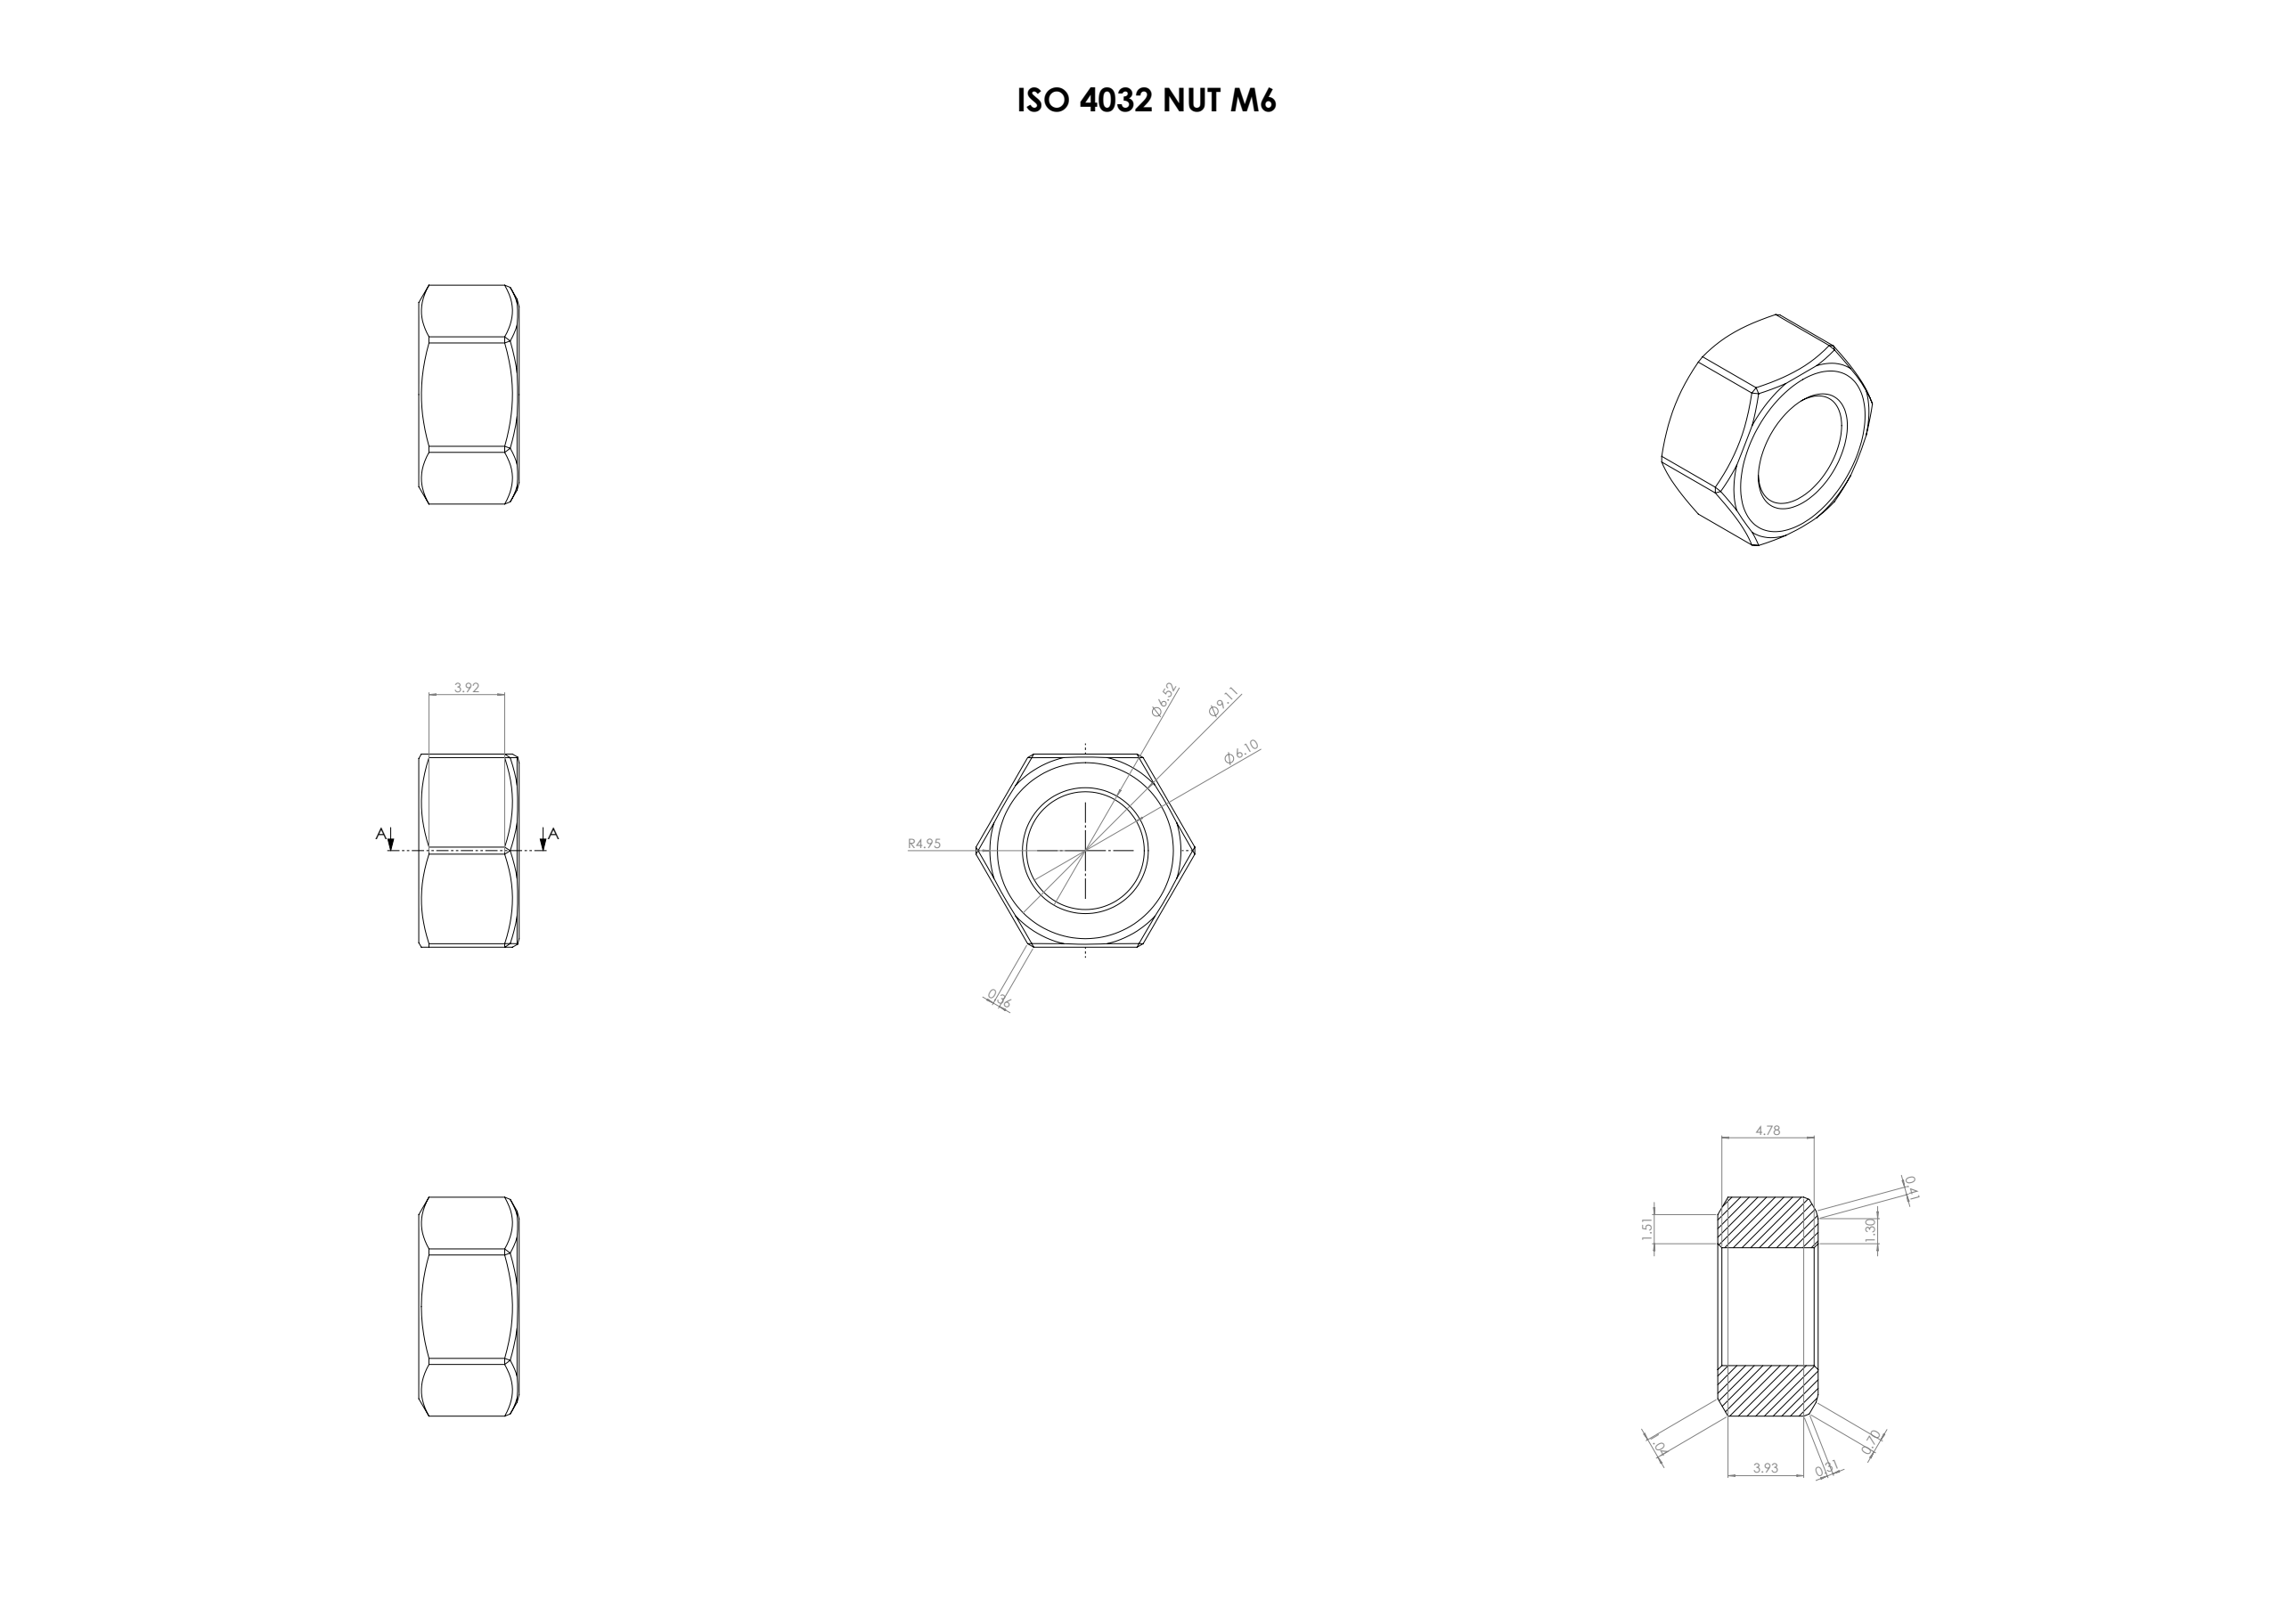
ISO-10303-21;
HEADER;
/* Generated by software containing ST-Developer
 * from STEP Tools, Inc. (www.steptools.com) 
 */

FILE_DESCRIPTION(
/* description */ (''),
/* implementation_level */ '2;1');

FILE_NAME(
/* name */ '08_ISO_4032_Nut_M6.step',
/* time_stamp */ '2026-10-21T02:03:06-07:00',
/* author */ (''),
/* organization */ (''),
/* preprocessor_version */ 'ST-DEVELOPER v20.2',
/* originating_system */ 'Autodesk Translation Framework v15.15.0.0',
/* authorisation */ '');

FILE_SCHEMA (('AUTOMOTIVE_DESIGN { 1 0 10303 214 3 1 1 }'));
ENDSEC;

DATA;
#10=MECHANICAL_DESIGN_GEOMETRIC_PRESENTATION_REPRESENTATION('',(#122),#38528);
#80=B_SPLINE_SURFACE_WITH_KNOTS('',3,3,((#33437,#33438,#33439,#33440,#33441),
(#33442,#33443,#33444,#33445,#33446),(#33447,#33448,#33449,#33450,#33451),
(#33452,#33453,#33454,#33455,#33456)),.UNSPECIFIED.,.F.,.F.,.F.,(4,4),(4,
1,4),(0.,1.),(0.0610870649866808,0.309114526274187,0.639817807990862),
 .UNSPECIFIED.);
#81=B_SPLINE_SURFACE_WITH_KNOTS('',3,3,((#33486,#33487,#33488,#33489,#33490),
(#33491,#33492,#33493,#33494,#33495),(#33496,#33497,#33498,#33499,#33500),
(#33501,#33502,#33503,#33504,#33505)),.UNSPECIFIED.,.F.,.F.,.F.,(4,4),(4,
1,4),(0.,1.),(0.0610870649866807,0.309114526274187,0.639817807990862),
 .UNSPECIFIED.);
#82=B_SPLINE_SURFACE_WITH_KNOTS('',3,3,((#33575,#33576,#33577,#33578,#33579),
(#33580,#33581,#33582,#33583,#33584),(#33585,#33586,#33587,#33588,#33589),
(#33590,#33591,#33592,#33593,#33594)),.UNSPECIFIED.,.F.,.F.,.F.,(4,4),(4,
1,4),(0.,1.),(0.061087064986681,0.309114526274187,0.639817807990862),
 .UNSPECIFIED.);
#83=B_SPLINE_SURFACE_WITH_KNOTS('',3,3,((#33668,#33669,#33670,#33671,#33672),
(#33673,#33674,#33675,#33676,#33677),(#33678,#33679,#33680,#33681,#33682),
(#33683,#33684,#33685,#33686,#33687)),.UNSPECIFIED.,.F.,.F.,.F.,(4,4),(4,
1,4),(0.,1.),(0.0610870649866801,0.309114526274187,0.639817807990862),
 .UNSPECIFIED.);
#84=B_SPLINE_SURFACE_WITH_KNOTS('',3,3,((#33701,#33702,#33703,#33704,#33705),
(#33706,#33707,#33708,#33709,#33710),(#33711,#33712,#33713,#33714,#33715),
(#33716,#33717,#33718,#33719,#33720)),.UNSPECIFIED.,.F.,.F.,.F.,(4,4),(4,
1,4),(0.,1.),(0.0610870649866807,0.391790346703356,0.639817807990862),
 .UNSPECIFIED.);
#85=B_SPLINE_SURFACE_WITH_KNOTS('',3,3,((#33742,#33743,#33744,#33745,#33746),
(#33747,#33748,#33749,#33750,#33751),(#33752,#33753,#33754,#33755,#33756),
(#33757,#33758,#33759,#33760,#33761)),.UNSPECIFIED.,.F.,.F.,.F.,(4,4),(4,
1,4),(0.,1.),(0.0610870649866804,0.309114526274187,0.639817807990861),
 .UNSPECIFIED.);
#98=SHAPE_REPRESENTATION_RELATIONSHIP('SRR','None',#38583,#110);
#110=ADVANCED_BREP_SHAPE_REPRESENTATION('',(#134),#38523);
#122=STYLED_ITEM('',(#38713),#134);
#134=MANIFOLD_SOLID_BREP('Body1',#17079);
#385=CYLINDRICAL_SURFACE('',#18726,3.05);
#719=B_SPLINE_CURVE_WITH_KNOTS('',3,(#33230,#33231,#33232,#33233,#33234,
#33235,#33236,#33237,#33238,#33239,#33240,#33241,#33242,#33243,#33244,#33245,
#33246,#33247,#33248),.UNSPECIFIED.,.F.,.F.,(4,3,3,3,3,3,4),(-0.113329393083273,
-0.0991044193051623,-0.0674458844185764,-0.061631000326846,-0.0331038403136512,
-0.00584534044920819,0.),.UNSPECIFIED.);
#720=B_SPLINE_CURVE_WITH_KNOTS('',3,(#33252,#33253,#33254,#33255,#33256,
#33257,#33258,#33259,#33260,#33261,#33262,#33263,#33264,#33265,#33266,#33267,
#33268,#33269,#33270,#33271,#33272,#33273,#33274,#33275,#33276,#33277,#33278,
#33279,#33280,#33281,#33282),.UNSPECIFIED.,.F.,.F.,(4,3,3,3,3,3,3,3,3,3,
4),(-0.226650511587635,-0.198574388081722,-0.170498264575808,-0.13944012666617,
-0.131476509591221,-0.0991044193051576,-0.0762723334429418,-0.0616310003268515,
-0.0331662800001561,-0.00604790654757715,0.),.UNSPECIFIED.);
#721=B_SPLINE_CURVE_WITH_KNOTS('',3,(#33286,#33287,#33288,#33289,#33290,
#33291,#33292,#33293,#33294,#33295,#33296,#33297,#33298,#33299,#33300,#33301,
#33302,#33303,#33304,#33305,#33306,#33307,#33308,#33309,#33310,#33311,#33312,
#33313,#33314,#33315,#33316),.UNSPECIFIED.,.F.,.F.,(4,3,3,3,3,3,3,3,3,3,
4),(-0.226650511587582,-0.198574388081676,-0.170498264575771,-0.13944012666705,
-0.131476509591215,-0.0991044193051536,-0.0762723334429342,-0.0616310003268419,
-0.0331662799998172,-0.00604790654743552,0.),.UNSPECIFIED.);
#722=B_SPLINE_CURVE_WITH_KNOTS('',3,(#33320,#33321,#33322,#33323,#33324,
#33325,#33326,#33327,#33328,#33329,#33330,#33331,#33332,#33333,#33334,#33335,
#33336,#33337,#33338,#33339,#33340,#33341,#33342,#33343,#33344,#33345,#33346,
#33347,#33348,#33349,#33350),.UNSPECIFIED.,.F.,.F.,(4,3,3,3,3,3,3,3,3,3,
4),(-0.226650511587584,-0.198574388081659,-0.170498264575734,-0.139440596738821,
-0.131476509591163,-0.0991044193051282,-0.0762723334429448,-0.0616310003268502,
-0.0331645723826234,-0.00604411953936661,0.),.UNSPECIFIED.);
#723=B_SPLINE_CURVE_WITH_KNOTS('',3,(#33354,#33355,#33356,#33357,#33358,
#33359,#33360,#33361,#33362,#33363,#33364,#33365,#33366,#33367,#33368,#33369,
#33370,#33371,#33372,#33373,#33374,#33375,#33376,#33377,#33378,#33379,#33380,
#33381,#33382,#33383,#33384),.UNSPECIFIED.,.F.,.F.,(4,3,3,3,3,3,3,3,3,3,
4),(-0.226650511587706,-0.198574388081775,-0.170498264575844,-0.139440126665696,
-0.131476509591268,-0.0991044193051773,-0.0762723334429522,-0.0616310003268415,
-0.0331662800006236,-0.00604790654845245,0.),.UNSPECIFIED.);
#724=B_SPLINE_CURVE_WITH_KNOTS('',3,(#33388,#33389,#33390,#33391,#33392,
#33393,#33394,#33395,#33396,#33397,#33398,#33399,#33400,#33401,#33402,#33403,
#33404,#33405,#33406,#33407,#33408,#33409,#33410,#33411,#33412,#33413,#33414,
#33415,#33416,#33417,#33418),.UNSPECIFIED.,.F.,.F.,(4,3,3,3,3,3,3,3,3,3,
4),(-0.226650511587727,-0.198574388081779,-0.170498264575831,-0.139440126665785,
-0.13147650959124,-0.0991044193051654,-0.0762723334429508,-0.0616310003268513,
-0.0331662799998889,-0.00604790654758933,0.),.UNSPECIFIED.);
#725=B_SPLINE_CURVE_WITH_KNOTS('',3,(#33421,#33422,#33423,#33424,#33425,
#33426,#33427,#33428,#33429,#33430,#33431,#33432,#33433,#33434,#33435,#33436),
 .UNSPECIFIED.,.F.,.F.,(4,3,3,3,3,4),(-0.226650511587688,-0.198574388081761,
-0.170498264575834,-0.150386414929284,-0.131476509591241,-0.113329393083273),
 .UNSPECIFIED.);
#726=B_SPLINE_CURVE_WITH_KNOTS('',3,(#33458,#33459,#33460,#33461),
 .UNSPECIFIED.,.F.,.F.,(4,4),(0.474834937773607,0.639817807990862),
 .UNSPECIFIED.);
#727=B_SPLINE_CURVE_WITH_KNOTS('',3,(#33463,#33464,#33465,#33466,#33467,
#33468),.UNSPECIFIED.,.F.,.F.,(4,2,4),(-0.0356915196979304,-0.0178436364936306,
0.),.UNSPECIFIED.);
#728=B_SPLINE_CURVE_WITH_KNOTS('',3,(#33470,#33471,#33472,#33473,#33474),
 .UNSPECIFIED.,.F.,.F.,(4,1,4),(-0.63803777562903,-0.309114526274187,-0.0628670973485611),
 .UNSPECIFIED.);
#729=B_SPLINE_CURVE_WITH_KNOTS('',3,(#33476,#33477,#33478,#33479,#33480,
#33481),.UNSPECIFIED.,.F.,.F.,(4,2,4),(-0.035691517766977,-0.0178476663798058,
0.),.UNSPECIFIED.);
#730=B_SPLINE_CURVE_WITH_KNOTS('',3,(#33482,#33483,#33484,#33485),
 .UNSPECIFIED.,.F.,.F.,(4,4),(0.0610870649866808,0.226069935203935),
 .UNSPECIFIED.);
#731=B_SPLINE_CURVE_WITH_KNOTS('',3,(#33507,#33508,#33509,#33510),
 .UNSPECIFIED.,.F.,.F.,(4,4),(0.474834937773608,0.639817807990862),
 .UNSPECIFIED.);
#732=B_SPLINE_CURVE_WITH_KNOTS('',3,(#33512,#33513,#33514,#33515,#33516,
#33517),.UNSPECIFIED.,.F.,.F.,(4,2,4),(-0.0356915197043745,-0.0178436364953559,
0.),.UNSPECIFIED.);
#733=B_SPLINE_CURVE_WITH_KNOTS('',3,(#33519,#33520,#33521,#33522,#33523),
 .UNSPECIFIED.,.F.,.F.,(4,1,4),(-0.638037775629031,-0.309114526274187,-0.062867097348561),
 .UNSPECIFIED.);
#734=B_SPLINE_CURVE_WITH_KNOTS('',3,(#33524,#33525,#33526,#33527,#33528,
#33529),.UNSPECIFIED.,.F.,.F.,(4,2,4),(-0.0356915177684809,-0.0178476663801996,
0.),.UNSPECIFIED.);
#735=B_SPLINE_CURVE_WITH_KNOTS('',3,(#33530,#33531,#33532,#33533),
 .UNSPECIFIED.,.F.,.F.,(4,4),(0.0610870649866807,0.226069935203935),
 .UNSPECIFIED.);
#736=B_SPLINE_CURVE_WITH_KNOTS('',3,(#33536,#33537,#33538,#33539),
 .UNSPECIFIED.,.F.,.F.,(4,4),(0.061087064986681,0.226069935203935),
 .UNSPECIFIED.);
#737=B_SPLINE_CURVE_WITH_KNOTS('',3,(#33542,#33543,#33544,#33545),
 .UNSPECIFIED.,.F.,.F.,(4,4),(0.0610870649866804,0.226069935203935),
 .UNSPECIFIED.);
#738=B_SPLINE_CURVE_WITH_KNOTS('',3,(#33546,#33547,#33548,#33549),
 .UNSPECIFIED.,.F.,.F.,(4,4),(0.474834937773607,0.639817807990862),
 .UNSPECIFIED.);
#739=B_SPLINE_CURVE_WITH_KNOTS('',3,(#33552,#33553,#33554,#33555),
 .UNSPECIFIED.,.F.,.F.,(4,4),(0.0610870649866807,0.226069935203935),
 .UNSPECIFIED.);
#740=B_SPLINE_CURVE_WITH_KNOTS('',3,(#33556,#33557,#33558,#33559),
 .UNSPECIFIED.,.F.,.F.,(4,4),(0.474834937773607,0.639817807990861),
 .UNSPECIFIED.);
#741=B_SPLINE_CURVE_WITH_KNOTS('',3,(#33562,#33563,#33564,#33565),
 .UNSPECIFIED.,.F.,.F.,(4,4),(0.0610870649866801,0.226069935203935),
 .UNSPECIFIED.);
#742=B_SPLINE_CURVE_WITH_KNOTS('',3,(#33566,#33567,#33568,#33569),
 .UNSPECIFIED.,.F.,.F.,(4,4),(0.474834937773608,0.639817807990862),
 .UNSPECIFIED.);
#743=B_SPLINE_CURVE_WITH_KNOTS('',3,(#33571,#33572,#33573,#33574),
 .UNSPECIFIED.,.F.,.F.,(4,4),(0.474834937773608,0.639817807990862),
 .UNSPECIFIED.);
#744=B_SPLINE_CURVE_WITH_KNOTS('',3,(#33596,#33597,#33598,#33599,#33600,
#33601),.UNSPECIFIED.,.F.,.F.,(4,2,4),(-0.0356915197030877,-0.0178436364955222,
0.),.UNSPECIFIED.);
#745=B_SPLINE_CURVE_WITH_KNOTS('',3,(#33603,#33604,#33605,#33606,#33607),
 .UNSPECIFIED.,.F.,.F.,(4,1,4),(-0.63803777562903,-0.309114526274187,-0.0628670973485611),
 .UNSPECIFIED.);
#746=B_SPLINE_CURVE_WITH_KNOTS('',3,(#33608,#33609,#33610,#33611,#33612,
#33613),.UNSPECIFIED.,.F.,.F.,(4,2,4),(-0.0356915177637329,-0.0178476663792099,
0.),.UNSPECIFIED.);
#747=B_SPLINE_CURVE_WITH_KNOTS('',3,(#33618,#33619,#33620,#33621,#33622,
#33623),.UNSPECIFIED.,.F.,.F.,(4,2,4),(-0.0356915177685627,-0.0178476663800234,
0.),.UNSPECIFIED.);
#748=B_SPLINE_CURVE_WITH_KNOTS('',3,(#33629,#33630,#33631,#33632,#33633,
#33634),.UNSPECIFIED.,.F.,.F.,(4,2,4),(-0.035691519698345,-0.0178436364936918,
0.),.UNSPECIFIED.);
#749=B_SPLINE_CURVE_WITH_KNOTS('',3,(#33636,#33637,#33638,#33639,#33640,
#33641),.UNSPECIFIED.,.F.,.F.,(4,2,4),(-0.0356915177661021,-0.0178476663801455,
0.),.UNSPECIFIED.);
#750=B_SPLINE_CURVE_WITH_KNOTS('',3,(#33646,#33647,#33648,#33649,#33650,
#33651),.UNSPECIFIED.,.F.,.F.,(4,2,4),(-0.0356915197010578,-0.0178436364947975,
0.),.UNSPECIFIED.);
#751=B_SPLINE_CURVE_WITH_KNOTS('',3,(#33654,#33655,#33656,#33657,#33658,
#33659),.UNSPECIFIED.,.F.,.F.,(4,2,4),(-0.0356915196998398,-0.0178436364940569,
0.),.UNSPECIFIED.);
#752=B_SPLINE_CURVE_WITH_KNOTS('',3,(#33661,#33662,#33663,#33664,#33665,
#33666),.UNSPECIFIED.,.F.,.F.,(4,2,4),(-0.0356915177634285,-0.0178476663777042,
0.),.UNSPECIFIED.);
#753=B_SPLINE_CURVE_WITH_KNOTS('',3,(#33688,#33689,#33690,#33691,#33692),
 .UNSPECIFIED.,.F.,.F.,(4,1,4),(-0.63803777562903,-0.309114526274187,-0.0628670973485611),
 .UNSPECIFIED.);
#754=B_SPLINE_CURVE_WITH_KNOTS('',3,(#33721,#33722,#33723,#33724,#33725),
 .UNSPECIFIED.,.F.,.F.,(4,1,4),(-0.638037775629031,-0.391790346703356,-0.0628670973485609),
 .UNSPECIFIED.);
#755=B_SPLINE_CURVE_WITH_KNOTS('',3,(#33762,#33763,#33764,#33765,#33766),
 .UNSPECIFIED.,.F.,.F.,(4,1,4),(-0.63803777562903,-0.309114526274187,-0.0628670973485611),
 .UNSPECIFIED.);
#1036=CONICAL_SURFACE('',#18723,3.155,0.785398163397449);
#1037=CONICAL_SURFACE('',#18730,3.155,0.785398163397448);
#1038=CONICAL_SURFACE('',#18734,4.75273145074145,1.30617281831714);
#1039=CONICAL_SURFACE('',#18741,5.41175134594813,1.04154930983939);
#1040=CONICAL_SURFACE('',#18742,5.41175134594813,1.04154930983939);
#1041=CONICAL_SURFACE('',#18743,5.41175134594813,1.04154930983939);
#1042=CONICAL_SURFACE('',#18744,5.41175134594813,1.04154930983939);
#1043=CONICAL_SURFACE('',#18745,5.41175134594813,1.04154930983939);
#1044=CONICAL_SURFACE('',#18746,5.41175134594813,1.04154930983939);
#1045=CONICAL_SURFACE('',#18762,5.41175134594813,1.04154930983939);
#1351=(
BOUNDED_CURVE()
B_SPLINE_CURVE(2,(#33696,#33697,#33698),.UNSPECIFIED.,.F.,.F.)
B_SPLINE_CURVE_WITH_KNOTS((3,3),(0.0914017655662012,0.12815983246024),
 .UNSPECIFIED.)
CURVE()
GEOMETRIC_REPRESENTATION_ITEM()
RATIONAL_B_SPLINE_CURVE((1.00900211770899,1.00952129238834,1.00900211770899))
REPRESENTATION_ITEM('')
);
#1352=(
BOUNDED_CURVE()
B_SPLINE_CURVE(2,(#33729,#33730,#33731),.UNSPECIFIED.,.F.,.F.)
B_SPLINE_CURVE_WITH_KNOTS((3,3),(0.091401765566201,0.12815983246024),
 .UNSPECIFIED.)
CURVE()
GEOMETRIC_REPRESENTATION_ITEM()
RATIONAL_B_SPLINE_CURVE((1.009002117709,1.00952129238836,1.009002117709))
REPRESENTATION_ITEM('')
);
#1353=(
BOUNDED_CURVE()
B_SPLINE_CURVE(2,(#33737,#33738,#33739),.UNSPECIFIED.,.F.,.F.)
B_SPLINE_CURVE_WITH_KNOTS((3,3),(0.0914017655662024,0.128159832460242),
 .UNSPECIFIED.)
CURVE()
GEOMETRIC_REPRESENTATION_ITEM()
RATIONAL_B_SPLINE_CURVE((1.00900211770901,1.00952129238837,1.00900211770901))
REPRESENTATION_ITEM('')
);
#1354=(
BOUNDED_CURVE()
B_SPLINE_CURVE(2,(#33770,#33771,#33772),.UNSPECIFIED.,.F.,.F.)
B_SPLINE_CURVE_WITH_KNOTS((3,3),(0.0914017655662023,0.128159832460241),
 .UNSPECIFIED.)
CURVE()
GEOMETRIC_REPRESENTATION_ITEM()
RATIONAL_B_SPLINE_CURVE((1.00900211770899,1.00952129238835,1.00900211770899))
REPRESENTATION_ITEM('')
);
#1355=(
BOUNDED_CURVE()
B_SPLINE_CURVE(2,(#33778,#33779,#33780),.UNSPECIFIED.,.F.,.F.)
B_SPLINE_CURVE_WITH_KNOTS((3,3),(0.091401765566202,0.128159832460241),
 .UNSPECIFIED.)
CURVE()
GEOMETRIC_REPRESENTATION_ITEM()
RATIONAL_B_SPLINE_CURVE((1.009002117709,1.00952129238836,1.009002117709))
REPRESENTATION_ITEM('')
);
#1356=(
BOUNDED_CURVE()
B_SPLINE_CURVE(2,(#33786,#33787,#33788),.UNSPECIFIED.,.F.,.F.)
B_SPLINE_CURVE_WITH_KNOTS((3,3),(0.0914017655662003,0.128159832460239),
 .UNSPECIFIED.)
CURVE()
GEOMETRIC_REPRESENTATION_ITEM()
RATIONAL_B_SPLINE_CURVE((1.009002117709,1.00952129238835,1.009002117709))
REPRESENTATION_ITEM('')
);
#1357=(
BOUNDED_CURVE()
B_SPLINE_CURVE(2,(#33792,#33793,#33794),.UNSPECIFIED.,.F.,.F.)
B_SPLINE_CURVE_WITH_KNOTS((3,3),(0.068123192861032,0.632781680116511),
 .UNSPECIFIED.)
CURVE()
GEOMETRIC_REPRESENTATION_ITEM()
RATIONAL_B_SPLINE_CURVE((1.03767852232438,1.17702201605488,1.03767852232437))
REPRESENTATION_ITEM('')
);
#1358=(
BOUNDED_CURVE()
B_SPLINE_CURVE(2,(#33796,#33797,#33798),.UNSPECIFIED.,.F.,.F.)
B_SPLINE_CURVE_WITH_KNOTS((3,3),(0.0681231928610322,0.632781680116511),
 .UNSPECIFIED.)
CURVE()
GEOMETRIC_REPRESENTATION_ITEM()
RATIONAL_B_SPLINE_CURVE((1.03767852232438,1.17702201605488,1.03767852232437))
REPRESENTATION_ITEM('')
);
#1359=(
BOUNDED_CURVE()
B_SPLINE_CURVE(2,(#33800,#33801,#33802),.UNSPECIFIED.,.F.,.F.)
B_SPLINE_CURVE_WITH_KNOTS((3,3),(0.0681231928610319,0.632781680116511),
 .UNSPECIFIED.)
CURVE()
GEOMETRIC_REPRESENTATION_ITEM()
RATIONAL_B_SPLINE_CURVE((1.03767852232438,1.17702201605488,1.03767852232438))
REPRESENTATION_ITEM('')
);
#1360=(
BOUNDED_CURVE()
B_SPLINE_CURVE(2,(#33806,#33807,#33808),.UNSPECIFIED.,.F.,.F.)
B_SPLINE_CURVE_WITH_KNOTS((3,3),(0.0681231928610319,0.350452436488771),
 .UNSPECIFIED.)
CURVE()
GEOMETRIC_REPRESENTATION_ITEM()
RATIONAL_B_SPLINE_CURVE((1.03767852232438,1.10735026918963,1.10735026918963))
REPRESENTATION_ITEM('')
);
#1361=(
BOUNDED_CURVE()
B_SPLINE_CURVE(2,(#33809,#33810,#33811),.UNSPECIFIED.,.F.,.F.)
B_SPLINE_CURVE_WITH_KNOTS((3,3),(0.068123192861032,0.632781680116511),
 .UNSPECIFIED.)
CURVE()
GEOMETRIC_REPRESENTATION_ITEM()
RATIONAL_B_SPLINE_CURVE((1.03767852232437,1.17702201605488,1.03767852232437))
REPRESENTATION_ITEM('')
);
#1362=(
BOUNDED_CURVE()
B_SPLINE_CURVE(2,(#33812,#33813,#33814),.UNSPECIFIED.,.F.,.F.)
B_SPLINE_CURVE_WITH_KNOTS((3,3),(0.0681231928610317,0.632781680116511),
 .UNSPECIFIED.)
CURVE()
GEOMETRIC_REPRESENTATION_ITEM()
RATIONAL_B_SPLINE_CURVE((1.03767852232438,1.17702201605488,1.03767852232438))
REPRESENTATION_ITEM('')
);
#1363=(
BOUNDED_CURVE()
B_SPLINE_CURVE(2,(#33815,#33816,#33817),.UNSPECIFIED.,.F.,.F.)
B_SPLINE_CURVE_WITH_KNOTS((3,3),(0.350452436488771,0.632781680116511),
 .UNSPECIFIED.)
CURVE()
GEOMETRIC_REPRESENTATION_ITEM()
RATIONAL_B_SPLINE_CURVE((1.10735026918963,1.10735026918963,1.03767852232438))
REPRESENTATION_ITEM('')
);
#1473=FACE_BOUND('',#4093,.T.);
#1474=FACE_BOUND('',#4096,.T.);
#2184=CIRCLE('',#18724,3.26);
#2185=CIRCLE('',#18725,3.05);
#2186=CIRCLE('',#18727,3.05);
#2187=CIRCLE('',#18729,4.76709676493043);
#2188=CIRCLE('',#18731,3.26);
#2189=CIRCLE('',#18733,4.55709676493043);
#2190=CIRCLE('',#18735,4.94836613655247);
#2191=CIRCLE('',#18736,4.94836613655247);
#2192=CIRCLE('',#18737,4.94836613655247);
#2193=CIRCLE('',#18738,4.94836613655247);
#2194=CIRCLE('',#18739,4.94836613655247);
#2195=CIRCLE('',#18740,4.94836613655247);
#3066=FACE_OUTER_BOUND('',#4090,.T.);
#3067=FACE_OUTER_BOUND('',#4091,.T.);
#3068=FACE_OUTER_BOUND('',#4092,.T.);
#3069=FACE_OUTER_BOUND('',#4094,.T.);
#3070=FACE_OUTER_BOUND('',#4095,.T.);
#3071=FACE_OUTER_BOUND('',#4097,.T.);
#3072=FACE_OUTER_BOUND('',#4098,.T.);
#3073=FACE_OUTER_BOUND('',#4099,.T.);
#3074=FACE_OUTER_BOUND('',#4100,.T.);
#3075=FACE_OUTER_BOUND('',#4101,.T.);
#3076=FACE_OUTER_BOUND('',#4102,.T.);
#3077=FACE_OUTER_BOUND('',#4103,.T.);
#3078=FACE_OUTER_BOUND('',#4104,.T.);
#3079=FACE_OUTER_BOUND('',#4105,.T.);
#3080=FACE_OUTER_BOUND('',#4106,.T.);
#3081=FACE_OUTER_BOUND('',#4107,.T.);
#3082=FACE_OUTER_BOUND('',#4108,.T.);
#3083=FACE_OUTER_BOUND('',#4109,.T.);
#3084=FACE_OUTER_BOUND('',#4110,.T.);
#3085=FACE_OUTER_BOUND('',#4111,.T.);
#3086=FACE_OUTER_BOUND('',#4112,.T.);
#3087=FACE_OUTER_BOUND('',#4113,.T.);
#3088=FACE_OUTER_BOUND('',#4114,.T.);
#3089=FACE_OUTER_BOUND('',#4115,.T.);
#3090=FACE_OUTER_BOUND('',#4116,.T.);
#3091=FACE_OUTER_BOUND('',#4117,.T.);
#3092=FACE_OUTER_BOUND('',#4118,.T.);
#3093=FACE_OUTER_BOUND('',#4119,.T.);
#3094=FACE_OUTER_BOUND('',#4120,.T.);
#3095=FACE_OUTER_BOUND('',#4121,.T.);
#3096=FACE_OUTER_BOUND('',#4122,.T.);
#3097=FACE_OUTER_BOUND('',#4123,.T.);
#3098=FACE_OUTER_BOUND('',#4124,.T.);
#3099=FACE_OUTER_BOUND('',#4125,.T.);
#3100=FACE_OUTER_BOUND('',#4126,.T.);
#3101=FACE_OUTER_BOUND('',#4127,.T.);
#3102=FACE_OUTER_BOUND('',#4128,.T.);
#4090=EDGE_LOOP('',(#14553,#14554,#14555,#14556));
#4091=EDGE_LOOP('',(#14557,#14558,#14559,#14560));
#4092=EDGE_LOOP('',(#14561));
#4093=EDGE_LOOP('',(#14562));
#4094=EDGE_LOOP('',(#14563,#14564,#14565,#14566));
#4095=EDGE_LOOP('',(#14567));
#4096=EDGE_LOOP('',(#14568));
#4097=EDGE_LOOP('',(#14569,#14570,#14571,#14572,#14573,#14574,#14575,#14576,
#14577,#14578,#14579,#14580,#14581,#14582,#14583,#14584));
#4098=EDGE_LOOP('',(#14585,#14586,#14587,#14588,#14589,#14590));
#4099=EDGE_LOOP('',(#14591,#14592,#14593,#14594,#14595,#14596));
#4100=EDGE_LOOP('',(#14597,#14598,#14599));
#4101=EDGE_LOOP('',(#14600,#14601,#14602));
#4102=EDGE_LOOP('',(#14603,#14604,#14605));
#4103=EDGE_LOOP('',(#14606,#14607,#14608));
#4104=EDGE_LOOP('',(#14609,#14610,#14611));
#4105=EDGE_LOOP('',(#14612,#14613,#14614));
#4106=EDGE_LOOP('',(#14615,#14616,#14617,#14618,#14619,#14620));
#4107=EDGE_LOOP('',(#14621,#14622,#14623));
#4108=EDGE_LOOP('',(#14624,#14625,#14626));
#4109=EDGE_LOOP('',(#14627,#14628,#14629));
#4110=EDGE_LOOP('',(#14630,#14631,#14632));
#4111=EDGE_LOOP('',(#14633,#14634,#14635));
#4112=EDGE_LOOP('',(#14636,#14637,#14638));
#4113=EDGE_LOOP('',(#14639,#14640,#14641,#14642,#14643,#14644));
#4114=EDGE_LOOP('',(#14645,#14646,#14647,#14648));
#4115=EDGE_LOOP('',(#14649,#14650,#14651,#14652,#14653,#14654,#14655));
#4116=EDGE_LOOP('',(#14656,#14657,#14658,#14659));
#4117=EDGE_LOOP('',(#14660,#14661,#14662,#14663));
#4118=EDGE_LOOP('',(#14664,#14665,#14666,#14667,#14668,#14669));
#4119=EDGE_LOOP('',(#14670,#14671,#14672,#14673));
#4120=EDGE_LOOP('',(#14674,#14675,#14676,#14677));
#4121=EDGE_LOOP('',(#14678,#14679,#14680,#14681));
#4122=EDGE_LOOP('',(#14682,#14683,#14684,#14685));
#4123=EDGE_LOOP('',(#14686,#14687,#14688,#14689));
#4124=EDGE_LOOP('',(#14690,#14691,#14692,#14693));
#4125=EDGE_LOOP('',(#14694,#14695,#14696,#14697,#14698,#14699,#14700,#14701,
#14702,#14703,#14704,#14705,#14706,#14707,#14708,#14709));
#4126=EDGE_LOOP('',(#14710,#14711,#14712,#14713));
#4127=EDGE_LOOP('',(#14714,#14715,#14716,#14717,#14718));
#4128=EDGE_LOOP('',(#14719,#14720,#14721,#14722));
#5032=LINE('',#33210,#6007);
#5033=LINE('',#33214,#6008);
#5034=LINE('',#33222,#6009);
#5035=LINE('',#33228,#6010);
#5036=LINE('',#33615,#6011);
#5037=LINE('',#33624,#6012);
#5038=LINE('',#33626,#6013);
#5039=LINE('',#33642,#6014);
#5040=LINE('',#33645,#6015);
#5041=LINE('',#33667,#6016);
#5042=LINE('',#33699,#6017);
#5043=LINE('',#33700,#6018);
#5044=LINE('',#33732,#6019);
#5045=LINE('',#33733,#6020);
#5046=LINE('',#33740,#6021);
#5047=LINE('',#33741,#6022);
#5048=LINE('',#33773,#6023);
#5049=LINE('',#33774,#6024);
#5050=LINE('',#33781,#6025);
#5051=LINE('',#33782,#6026);
#5052=LINE('',#33789,#6027);
#5053=LINE('',#33790,#6028);
#5054=LINE('',#33805,#6029);
#6007=VECTOR('',#22782,3.155);
#6008=VECTOR('',#22787,3.05);
#6009=VECTOR('',#22798,3.155);
#6010=VECTOR('',#22805,4.75273145074145);
#6011=VECTOR('',#22832,10.);
#6012=VECTOR('',#22835,10.);
#6013=VECTOR('',#22838,10.);
#6014=VECTOR('',#22841,10.);
#6015=VECTOR('',#22844,10.);
#6016=VECTOR('',#22847,10.);
#6017=VECTOR('',#22850,10.);
#6018=VECTOR('',#22851,10.);
#6019=VECTOR('',#22854,10.);
#6020=VECTOR('',#22855,10.);
#6021=VECTOR('',#22858,10.);
#6022=VECTOR('',#22859,10.);
#6023=VECTOR('',#22862,10.);
#6024=VECTOR('',#22863,10.);
#6025=VECTOR('',#22866,10.);
#6026=VECTOR('',#22867,10.);
#6027=VECTOR('',#22870,10.);
#6028=VECTOR('',#22871,10.);
#6029=VECTOR('',#22880,5.41175134594813);
#7535=VERTEX_POINT('',#33207);
#7536=VERTEX_POINT('',#33209);
#7537=VERTEX_POINT('',#33213);
#7538=VERTEX_POINT('',#33217);
#7539=VERTEX_POINT('',#33220);
#7540=VERTEX_POINT('',#33224);
#7541=VERTEX_POINT('',#33227);
#7542=VERTEX_POINT('',#33229);
#7543=VERTEX_POINT('',#33249);
#7544=VERTEX_POINT('',#33251);
#7545=VERTEX_POINT('',#33283);
#7546=VERTEX_POINT('',#33285);
#7547=VERTEX_POINT('',#33317);
#7548=VERTEX_POINT('',#33319);
#7549=VERTEX_POINT('',#33351);
#7550=VERTEX_POINT('',#33353);
#7551=VERTEX_POINT('',#33385);
#7552=VERTEX_POINT('',#33387);
#7553=VERTEX_POINT('',#33419);
#7554=VERTEX_POINT('',#33457);
#7555=VERTEX_POINT('',#33462);
#7556=VERTEX_POINT('',#33469);
#7557=VERTEX_POINT('',#33475);
#7558=VERTEX_POINT('',#33506);
#7559=VERTEX_POINT('',#33511);
#7560=VERTEX_POINT('',#33518);
#7561=VERTEX_POINT('',#33541);
#7562=VERTEX_POINT('',#33551);
#7563=VERTEX_POINT('',#33561);
#7564=VERTEX_POINT('',#33595);
#7565=VERTEX_POINT('',#33602);
#7566=VERTEX_POINT('',#33617);
#7567=VERTEX_POINT('',#33628);
#7568=VERTEX_POINT('',#33635);
#7569=VERTEX_POINT('',#33644);
#7570=VERTEX_POINT('',#33653);
#7571=VERTEX_POINT('',#33660);
#7572=VERTEX_POINT('',#33694);
#7573=VERTEX_POINT('',#33695);
#7574=VERTEX_POINT('',#33727);
#7575=VERTEX_POINT('',#33728);
#7576=VERTEX_POINT('',#33735);
#7577=VERTEX_POINT('',#33736);
#7578=VERTEX_POINT('',#33768);
#7579=VERTEX_POINT('',#33769);
#7580=VERTEX_POINT('',#33776);
#7581=VERTEX_POINT('',#33777);
#7582=VERTEX_POINT('',#33784);
#7583=VERTEX_POINT('',#33785);
#7584=VERTEX_POINT('',#33804);
#9928=EDGE_CURVE('',#7535,#7535,#2184,.T.);
#9929=EDGE_CURVE('',#7535,#7536,#5032,.T.);
#9930=EDGE_CURVE('',#7536,#7536,#2185,.T.);
#9931=EDGE_CURVE('',#7536,#7537,#5033,.T.);
#9932=EDGE_CURVE('',#7537,#7537,#2186,.T.);
#9933=EDGE_CURVE('',#7538,#7538,#2187,.T.);
#9934=EDGE_CURVE('',#7539,#7539,#2188,.T.);
#9935=EDGE_CURVE('',#7539,#7537,#5034,.T.);
#9936=EDGE_CURVE('',#7540,#7540,#2189,.T.);
#9937=EDGE_CURVE('',#7540,#7541,#5035,.T.);
#9938=EDGE_CURVE('',#7541,#7542,#719,.T.);
#9939=EDGE_CURVE('',#7542,#7543,#2190,.T.);
#9940=EDGE_CURVE('',#7543,#7544,#720,.T.);
#9941=EDGE_CURVE('',#7544,#7545,#2191,.T.);
#9942=EDGE_CURVE('',#7545,#7546,#721,.T.);
#9943=EDGE_CURVE('',#7546,#7547,#2192,.T.);
#9944=EDGE_CURVE('',#7547,#7548,#722,.T.);
#9945=EDGE_CURVE('',#7548,#7549,#2193,.T.);
#9946=EDGE_CURVE('',#7549,#7550,#723,.T.);
#9947=EDGE_CURVE('',#7550,#7551,#2194,.T.);
#9948=EDGE_CURVE('',#7551,#7552,#724,.T.);
#9949=EDGE_CURVE('',#7552,#7553,#2195,.T.);
#9950=EDGE_CURVE('',#7553,#7541,#725,.T.);
#9951=EDGE_CURVE('',#7549,#7554,#726,.T.);
#9952=EDGE_CURVE('',#7554,#7555,#727,.F.);
#9953=EDGE_CURVE('',#7555,#7556,#728,.T.);
#9954=EDGE_CURVE('',#7556,#7557,#729,.F.);
#9955=EDGE_CURVE('',#7557,#7550,#730,.T.);
#9956=EDGE_CURVE('',#7547,#7558,#731,.T.);
#9957=EDGE_CURVE('',#7558,#7559,#732,.F.);
#9958=EDGE_CURVE('',#7559,#7560,#733,.T.);
#9959=EDGE_CURVE('',#7560,#7554,#734,.F.);
#9960=EDGE_CURVE('',#7554,#7548,#735,.T.);
#9961=EDGE_CURVE('',#7558,#7546,#736,.T.);
#9962=EDGE_CURVE('',#7561,#7544,#737,.T.);
#9963=EDGE_CURVE('',#7545,#7561,#738,.T.);
#9964=EDGE_CURVE('',#7562,#7542,#739,.T.);
#9965=EDGE_CURVE('',#7543,#7562,#740,.T.);
#9966=EDGE_CURVE('',#7563,#7552,#741,.T.);
#9967=EDGE_CURVE('',#7553,#7563,#742,.T.);
#9968=EDGE_CURVE('',#7551,#7557,#743,.T.);
#9969=EDGE_CURVE('',#7561,#7564,#744,.F.);
#9970=EDGE_CURVE('',#7564,#7565,#745,.T.);
#9971=EDGE_CURVE('',#7565,#7558,#746,.F.);
#9972=EDGE_CURVE('',#7559,#7565,#5036,.T.);
#9973=EDGE_CURVE('',#7566,#7561,#747,.F.);
#9974=EDGE_CURVE('',#7564,#7566,#5037,.T.);
#9975=EDGE_CURVE('',#7555,#7560,#5038,.T.);
#9976=EDGE_CURVE('',#7562,#7567,#748,.F.);
#9977=EDGE_CURVE('',#7568,#7562,#749,.F.);
#9978=EDGE_CURVE('',#7567,#7568,#5039,.T.);
#9979=EDGE_CURVE('',#7569,#7556,#5040,.T.);
#9980=EDGE_CURVE('',#7557,#7569,#750,.F.);
#9981=EDGE_CURVE('',#7563,#7570,#751,.F.);
#9982=EDGE_CURVE('',#7571,#7563,#752,.F.);
#9983=EDGE_CURVE('',#7570,#7571,#5041,.T.);
#9984=EDGE_CURVE('',#7569,#7571,#753,.T.);
#9985=EDGE_CURVE('',#7572,#7573,#1351,.T.);
#9986=EDGE_CURVE('',#7573,#7570,#5042,.T.);
#9987=EDGE_CURVE('',#7571,#7572,#5043,.T.);
#9988=EDGE_CURVE('',#7570,#7568,#754,.T.);
#9989=EDGE_CURVE('',#7574,#7575,#1352,.T.);
#9990=EDGE_CURVE('',#7575,#7569,#5044,.T.);
#9991=EDGE_CURVE('',#7556,#7574,#5045,.T.);
#9992=EDGE_CURVE('',#7576,#7577,#1353,.T.);
#9993=EDGE_CURVE('',#7577,#7567,#5046,.T.);
#9994=EDGE_CURVE('',#7568,#7576,#5047,.T.);
#9995=EDGE_CURVE('',#7567,#7566,#755,.T.);
#9996=EDGE_CURVE('',#7578,#7579,#1354,.T.);
#9997=EDGE_CURVE('',#7579,#7555,#5048,.T.);
#9998=EDGE_CURVE('',#7560,#7578,#5049,.T.);
#9999=EDGE_CURVE('',#7580,#7581,#1355,.T.);
#10000=EDGE_CURVE('',#7581,#7564,#5050,.T.);
#10001=EDGE_CURVE('',#7566,#7580,#5051,.T.);
#10002=EDGE_CURVE('',#7582,#7583,#1356,.T.);
#10003=EDGE_CURVE('',#7583,#7559,#5052,.T.);
#10004=EDGE_CURVE('',#7565,#7582,#5053,.T.);
#10005=EDGE_CURVE('',#7579,#7574,#1357,.T.);
#10006=EDGE_CURVE('',#7583,#7578,#1358,.T.);
#10007=EDGE_CURVE('',#7581,#7582,#1359,.T.);
#10008=EDGE_CURVE('',#7538,#7584,#5054,.T.);
#10009=EDGE_CURVE('',#7573,#7584,#1360,.T.);
#10010=EDGE_CURVE('',#7575,#7572,#1361,.T.);
#10011=EDGE_CURVE('',#7577,#7580,#1362,.T.);
#10012=EDGE_CURVE('',#7584,#7576,#1363,.T.);
#14553=ORIENTED_EDGE('',*,*,#9928,.T.);
#14554=ORIENTED_EDGE('',*,*,#9929,.T.);
#14555=ORIENTED_EDGE('',*,*,#9930,.T.);
#14556=ORIENTED_EDGE('',*,*,#9929,.F.);
#14557=ORIENTED_EDGE('',*,*,#9930,.F.);
#14558=ORIENTED_EDGE('',*,*,#9931,.T.);
#14559=ORIENTED_EDGE('',*,*,#9932,.F.);
#14560=ORIENTED_EDGE('',*,*,#9931,.F.);
#14561=ORIENTED_EDGE('',*,*,#9933,.T.);
#14562=ORIENTED_EDGE('',*,*,#9928,.F.);
#14563=ORIENTED_EDGE('',*,*,#9934,.T.);
#14564=ORIENTED_EDGE('',*,*,#9935,.T.);
#14565=ORIENTED_EDGE('',*,*,#9932,.T.);
#14566=ORIENTED_EDGE('',*,*,#9935,.F.);
#14567=ORIENTED_EDGE('',*,*,#9936,.F.);
#14568=ORIENTED_EDGE('',*,*,#9934,.F.);
#14569=ORIENTED_EDGE('',*,*,#9936,.T.);
#14570=ORIENTED_EDGE('',*,*,#9937,.T.);
#14571=ORIENTED_EDGE('',*,*,#9938,.T.);
#14572=ORIENTED_EDGE('',*,*,#9939,.T.);
#14573=ORIENTED_EDGE('',*,*,#9940,.T.);
#14574=ORIENTED_EDGE('',*,*,#9941,.T.);
#14575=ORIENTED_EDGE('',*,*,#9942,.T.);
#14576=ORIENTED_EDGE('',*,*,#9943,.T.);
#14577=ORIENTED_EDGE('',*,*,#9944,.T.);
#14578=ORIENTED_EDGE('',*,*,#9945,.T.);
#14579=ORIENTED_EDGE('',*,*,#9946,.T.);
#14580=ORIENTED_EDGE('',*,*,#9947,.T.);
#14581=ORIENTED_EDGE('',*,*,#9948,.T.);
#14582=ORIENTED_EDGE('',*,*,#9949,.T.);
#14583=ORIENTED_EDGE('',*,*,#9950,.T.);
#14584=ORIENTED_EDGE('',*,*,#9937,.F.);
#14585=ORIENTED_EDGE('',*,*,#9946,.F.);
#14586=ORIENTED_EDGE('',*,*,#9951,.T.);
#14587=ORIENTED_EDGE('',*,*,#9952,.T.);
#14588=ORIENTED_EDGE('',*,*,#9953,.T.);
#14589=ORIENTED_EDGE('',*,*,#9954,.T.);
#14590=ORIENTED_EDGE('',*,*,#9955,.T.);
#14591=ORIENTED_EDGE('',*,*,#9944,.F.);
#14592=ORIENTED_EDGE('',*,*,#9956,.T.);
#14593=ORIENTED_EDGE('',*,*,#9957,.T.);
#14594=ORIENTED_EDGE('',*,*,#9958,.T.);
#14595=ORIENTED_EDGE('',*,*,#9959,.T.);
#14596=ORIENTED_EDGE('',*,*,#9960,.T.);
#14597=ORIENTED_EDGE('',*,*,#9945,.F.);
#14598=ORIENTED_EDGE('',*,*,#9960,.F.);
#14599=ORIENTED_EDGE('',*,*,#9951,.F.);
#14600=ORIENTED_EDGE('',*,*,#9943,.F.);
#14601=ORIENTED_EDGE('',*,*,#9961,.F.);
#14602=ORIENTED_EDGE('',*,*,#9956,.F.);
#14603=ORIENTED_EDGE('',*,*,#9941,.F.);
#14604=ORIENTED_EDGE('',*,*,#9962,.F.);
#14605=ORIENTED_EDGE('',*,*,#9963,.F.);
#14606=ORIENTED_EDGE('',*,*,#9939,.F.);
#14607=ORIENTED_EDGE('',*,*,#9964,.F.);
#14608=ORIENTED_EDGE('',*,*,#9965,.F.);
#14609=ORIENTED_EDGE('',*,*,#9949,.F.);
#14610=ORIENTED_EDGE('',*,*,#9966,.F.);
#14611=ORIENTED_EDGE('',*,*,#9967,.F.);
#14612=ORIENTED_EDGE('',*,*,#9947,.F.);
#14613=ORIENTED_EDGE('',*,*,#9955,.F.);
#14614=ORIENTED_EDGE('',*,*,#9968,.F.);
#14615=ORIENTED_EDGE('',*,*,#9942,.F.);
#14616=ORIENTED_EDGE('',*,*,#9963,.T.);
#14617=ORIENTED_EDGE('',*,*,#9969,.T.);
#14618=ORIENTED_EDGE('',*,*,#9970,.T.);
#14619=ORIENTED_EDGE('',*,*,#9971,.T.);
#14620=ORIENTED_EDGE('',*,*,#9961,.T.);
#14621=ORIENTED_EDGE('',*,*,#9972,.F.);
#14622=ORIENTED_EDGE('',*,*,#9957,.F.);
#14623=ORIENTED_EDGE('',*,*,#9971,.F.);
#14624=ORIENTED_EDGE('',*,*,#9969,.F.);
#14625=ORIENTED_EDGE('',*,*,#9973,.F.);
#14626=ORIENTED_EDGE('',*,*,#9974,.F.);
#14627=ORIENTED_EDGE('',*,*,#9975,.F.);
#14628=ORIENTED_EDGE('',*,*,#9952,.F.);
#14629=ORIENTED_EDGE('',*,*,#9959,.F.);
#14630=ORIENTED_EDGE('',*,*,#9976,.F.);
#14631=ORIENTED_EDGE('',*,*,#9977,.F.);
#14632=ORIENTED_EDGE('',*,*,#9978,.F.);
#14633=ORIENTED_EDGE('',*,*,#9979,.F.);
#14634=ORIENTED_EDGE('',*,*,#9980,.F.);
#14635=ORIENTED_EDGE('',*,*,#9954,.F.);
#14636=ORIENTED_EDGE('',*,*,#9981,.F.);
#14637=ORIENTED_EDGE('',*,*,#9982,.F.);
#14638=ORIENTED_EDGE('',*,*,#9983,.F.);
#14639=ORIENTED_EDGE('',*,*,#9948,.F.);
#14640=ORIENTED_EDGE('',*,*,#9968,.T.);
#14641=ORIENTED_EDGE('',*,*,#9980,.T.);
#14642=ORIENTED_EDGE('',*,*,#9984,.T.);
#14643=ORIENTED_EDGE('',*,*,#9982,.T.);
#14644=ORIENTED_EDGE('',*,*,#9966,.T.);
#14645=ORIENTED_EDGE('',*,*,#9985,.T.);
#14646=ORIENTED_EDGE('',*,*,#9986,.T.);
#14647=ORIENTED_EDGE('',*,*,#9983,.T.);
#14648=ORIENTED_EDGE('',*,*,#9987,.T.);
#14649=ORIENTED_EDGE('',*,*,#9950,.F.);
#14650=ORIENTED_EDGE('',*,*,#9967,.T.);
#14651=ORIENTED_EDGE('',*,*,#9981,.T.);
#14652=ORIENTED_EDGE('',*,*,#9988,.T.);
#14653=ORIENTED_EDGE('',*,*,#9977,.T.);
#14654=ORIENTED_EDGE('',*,*,#9964,.T.);
#14655=ORIENTED_EDGE('',*,*,#9938,.F.);
#14656=ORIENTED_EDGE('',*,*,#9989,.T.);
#14657=ORIENTED_EDGE('',*,*,#9990,.T.);
#14658=ORIENTED_EDGE('',*,*,#9979,.T.);
#14659=ORIENTED_EDGE('',*,*,#9991,.T.);
#14660=ORIENTED_EDGE('',*,*,#9992,.T.);
#14661=ORIENTED_EDGE('',*,*,#9993,.T.);
#14662=ORIENTED_EDGE('',*,*,#9978,.T.);
#14663=ORIENTED_EDGE('',*,*,#9994,.T.);
#14664=ORIENTED_EDGE('',*,*,#9940,.F.);
#14665=ORIENTED_EDGE('',*,*,#9965,.T.);
#14666=ORIENTED_EDGE('',*,*,#9976,.T.);
#14667=ORIENTED_EDGE('',*,*,#9995,.T.);
#14668=ORIENTED_EDGE('',*,*,#9973,.T.);
#14669=ORIENTED_EDGE('',*,*,#9962,.T.);
#14670=ORIENTED_EDGE('',*,*,#9996,.T.);
#14671=ORIENTED_EDGE('',*,*,#9997,.T.);
#14672=ORIENTED_EDGE('',*,*,#9975,.T.);
#14673=ORIENTED_EDGE('',*,*,#9998,.T.);
#14674=ORIENTED_EDGE('',*,*,#9999,.T.);
#14675=ORIENTED_EDGE('',*,*,#10000,.T.);
#14676=ORIENTED_EDGE('',*,*,#9974,.T.);
#14677=ORIENTED_EDGE('',*,*,#10001,.T.);
#14678=ORIENTED_EDGE('',*,*,#10002,.T.);
#14679=ORIENTED_EDGE('',*,*,#10003,.T.);
#14680=ORIENTED_EDGE('',*,*,#9972,.T.);
#14681=ORIENTED_EDGE('',*,*,#10004,.T.);
#14682=ORIENTED_EDGE('',*,*,#9991,.F.);
#14683=ORIENTED_EDGE('',*,*,#9953,.F.);
#14684=ORIENTED_EDGE('',*,*,#9997,.F.);
#14685=ORIENTED_EDGE('',*,*,#10005,.T.);
#14686=ORIENTED_EDGE('',*,*,#9998,.F.);
#14687=ORIENTED_EDGE('',*,*,#9958,.F.);
#14688=ORIENTED_EDGE('',*,*,#10003,.F.);
#14689=ORIENTED_EDGE('',*,*,#10006,.T.);
#14690=ORIENTED_EDGE('',*,*,#10004,.F.);
#14691=ORIENTED_EDGE('',*,*,#9970,.F.);
#14692=ORIENTED_EDGE('',*,*,#10000,.F.);
#14693=ORIENTED_EDGE('',*,*,#10007,.T.);
#14694=ORIENTED_EDGE('',*,*,#9933,.F.);
#14695=ORIENTED_EDGE('',*,*,#10008,.T.);
#14696=ORIENTED_EDGE('',*,*,#10009,.F.);
#14697=ORIENTED_EDGE('',*,*,#9985,.F.);
#14698=ORIENTED_EDGE('',*,*,#10010,.F.);
#14699=ORIENTED_EDGE('',*,*,#9989,.F.);
#14700=ORIENTED_EDGE('',*,*,#10005,.F.);
#14701=ORIENTED_EDGE('',*,*,#9996,.F.);
#14702=ORIENTED_EDGE('',*,*,#10006,.F.);
#14703=ORIENTED_EDGE('',*,*,#10002,.F.);
#14704=ORIENTED_EDGE('',*,*,#10007,.F.);
#14705=ORIENTED_EDGE('',*,*,#9999,.F.);
#14706=ORIENTED_EDGE('',*,*,#10011,.F.);
#14707=ORIENTED_EDGE('',*,*,#9992,.F.);
#14708=ORIENTED_EDGE('',*,*,#10012,.F.);
#14709=ORIENTED_EDGE('',*,*,#10008,.F.);
#14710=ORIENTED_EDGE('',*,*,#9993,.F.);
#14711=ORIENTED_EDGE('',*,*,#10011,.T.);
#14712=ORIENTED_EDGE('',*,*,#10001,.F.);
#14713=ORIENTED_EDGE('',*,*,#9995,.F.);
#14714=ORIENTED_EDGE('',*,*,#9986,.F.);
#14715=ORIENTED_EDGE('',*,*,#10009,.T.);
#14716=ORIENTED_EDGE('',*,*,#10012,.T.);
#14717=ORIENTED_EDGE('',*,*,#9994,.F.);
#14718=ORIENTED_EDGE('',*,*,#9988,.F.);
#14719=ORIENTED_EDGE('',*,*,#9990,.F.);
#14720=ORIENTED_EDGE('',*,*,#10010,.T.);
#14721=ORIENTED_EDGE('',*,*,#9987,.F.);
#14722=ORIENTED_EDGE('',*,*,#9984,.F.);
#15962=PLANE('',#18728);
#15963=PLANE('',#18732);
#15964=PLANE('',#18747);
#15965=PLANE('',#18748);
#15966=PLANE('',#18749);
#15967=PLANE('',#18750);
#15968=PLANE('',#18751);
#15969=PLANE('',#18752);
#15970=PLANE('',#18753);
#15971=PLANE('',#18754);
#15972=PLANE('',#18755);
#15973=PLANE('',#18756);
#15974=PLANE('',#18757);
#15975=PLANE('',#18758);
#15976=PLANE('',#18759);
#15977=PLANE('',#18760);
#15978=PLANE('',#18761);
#15979=PLANE('',#18763);
#15980=PLANE('',#18764);
#15981=PLANE('',#18765);
#16875=ADVANCED_FACE('',(#3066),#1036,.F.);
#16876=ADVANCED_FACE('',(#3067),#385,.F.);
#16877=ADVANCED_FACE('',(#3068,#1473),#15962,.F.);
#16878=ADVANCED_FACE('',(#3069),#1037,.F.);
#16879=ADVANCED_FACE('',(#3070,#1474),#15963,.T.);
#16880=ADVANCED_FACE('',(#3071),#1038,.T.);
#16881=ADVANCED_FACE('',(#3072),#80,.T.);
#16882=ADVANCED_FACE('',(#3073),#81,.T.);
#16883=ADVANCED_FACE('',(#3074),#1039,.T.);
#16884=ADVANCED_FACE('',(#3075),#1040,.T.);
#16885=ADVANCED_FACE('',(#3076),#1041,.T.);
#16886=ADVANCED_FACE('',(#3077),#1042,.T.);
#16887=ADVANCED_FACE('',(#3078),#1043,.T.);
#16888=ADVANCED_FACE('',(#3079),#1044,.T.);
#16889=ADVANCED_FACE('',(#3080),#82,.T.);
#16890=ADVANCED_FACE('',(#3081),#15964,.T.);
#16891=ADVANCED_FACE('',(#3082),#15965,.T.);
#16892=ADVANCED_FACE('',(#3083),#15966,.T.);
#16893=ADVANCED_FACE('',(#3084),#15967,.T.);
#16894=ADVANCED_FACE('',(#3085),#15968,.T.);
#16895=ADVANCED_FACE('',(#3086),#15969,.T.);
#16896=ADVANCED_FACE('',(#3087),#83,.T.);
#16897=ADVANCED_FACE('',(#3088),#15970,.T.);
#16898=ADVANCED_FACE('',(#3089),#84,.T.);
#16899=ADVANCED_FACE('',(#3090),#15971,.T.);
#16900=ADVANCED_FACE('',(#3091),#15972,.T.);
#16901=ADVANCED_FACE('',(#3092),#85,.T.);
#16902=ADVANCED_FACE('',(#3093),#15973,.T.);
#16903=ADVANCED_FACE('',(#3094),#15974,.T.);
#16904=ADVANCED_FACE('',(#3095),#15975,.T.);
#16905=ADVANCED_FACE('',(#3096),#15976,.T.);
#16906=ADVANCED_FACE('',(#3097),#15977,.T.);
#16907=ADVANCED_FACE('',(#3098),#15978,.T.);
#16908=ADVANCED_FACE('',(#3099),#1045,.T.);
#16909=ADVANCED_FACE('',(#3100),#15979,.T.);
#16910=ADVANCED_FACE('',(#3101),#15980,.T.);
#16911=ADVANCED_FACE('',(#3102),#15981,.T.);
#17079=CLOSED_SHELL('',(#16875,#16876,#16877,#16878,#16879,#16880,#16881,
#16882,#16883,#16884,#16885,#16886,#16887,#16888,#16889,#16890,#16891,#16892,
#16893,#16894,#16895,#16896,#16897,#16898,#16899,#16900,#16901,#16902,#16903,
#16904,#16905,#16906,#16907,#16908,#16909,#16910,#16911));
#18722=AXIS2_PLACEMENT_3D('',#33205,#22776,#22777);
#18723=AXIS2_PLACEMENT_3D('',#33206,#22778,#22779);
#18724=AXIS2_PLACEMENT_3D('',#33208,#22780,#22781);
#18725=AXIS2_PLACEMENT_3D('',#33211,#22783,#22784);
#18726=AXIS2_PLACEMENT_3D('',#33212,#22785,#22786);
#18727=AXIS2_PLACEMENT_3D('',#33215,#22788,#22789);
#18728=AXIS2_PLACEMENT_3D('',#33216,#22790,#22791);
#18729=AXIS2_PLACEMENT_3D('',#33218,#22792,#22793);
#18730=AXIS2_PLACEMENT_3D('',#33219,#22794,#22795);
#18731=AXIS2_PLACEMENT_3D('',#33221,#22796,#22797);
#18732=AXIS2_PLACEMENT_3D('',#33223,#22799,#22800);
#18733=AXIS2_PLACEMENT_3D('',#33225,#22801,#22802);
#18734=AXIS2_PLACEMENT_3D('',#33226,#22803,#22804);
#18735=AXIS2_PLACEMENT_3D('',#33250,#22806,#22807);
#18736=AXIS2_PLACEMENT_3D('',#33284,#22808,#22809);
#18737=AXIS2_PLACEMENT_3D('',#33318,#22810,#22811);
#18738=AXIS2_PLACEMENT_3D('',#33352,#22812,#22813);
#18739=AXIS2_PLACEMENT_3D('',#33386,#22814,#22815);
#18740=AXIS2_PLACEMENT_3D('',#33420,#22816,#22817);
#18741=AXIS2_PLACEMENT_3D('',#33534,#22818,#22819);
#18742=AXIS2_PLACEMENT_3D('',#33535,#22820,#22821);
#18743=AXIS2_PLACEMENT_3D('',#33540,#22822,#22823);
#18744=AXIS2_PLACEMENT_3D('',#33550,#22824,#22825);
#18745=AXIS2_PLACEMENT_3D('',#33560,#22826,#22827);
#18746=AXIS2_PLACEMENT_3D('',#33570,#22828,#22829);
#18747=AXIS2_PLACEMENT_3D('',#33614,#22830,#22831);
#18748=AXIS2_PLACEMENT_3D('',#33616,#22833,#22834);
#18749=AXIS2_PLACEMENT_3D('',#33625,#22836,#22837);
#18750=AXIS2_PLACEMENT_3D('',#33627,#22839,#22840);
#18751=AXIS2_PLACEMENT_3D('',#33643,#22842,#22843);
#18752=AXIS2_PLACEMENT_3D('',#33652,#22845,#22846);
#18753=AXIS2_PLACEMENT_3D('',#33693,#22848,#22849);
#18754=AXIS2_PLACEMENT_3D('',#33726,#22852,#22853);
#18755=AXIS2_PLACEMENT_3D('',#33734,#22856,#22857);
#18756=AXIS2_PLACEMENT_3D('',#33767,#22860,#22861);
#18757=AXIS2_PLACEMENT_3D('',#33775,#22864,#22865);
#18758=AXIS2_PLACEMENT_3D('',#33783,#22868,#22869);
#18759=AXIS2_PLACEMENT_3D('',#33791,#22872,#22873);
#18760=AXIS2_PLACEMENT_3D('',#33795,#22874,#22875);
#18761=AXIS2_PLACEMENT_3D('',#33799,#22876,#22877);
#18762=AXIS2_PLACEMENT_3D('',#33803,#22878,#22879);
#18763=AXIS2_PLACEMENT_3D('',#33818,#22881,#22882);
#18764=AXIS2_PLACEMENT_3D('',#33819,#22883,#22884);
#18765=AXIS2_PLACEMENT_3D('',#33820,#22885,#22886);
#22776=DIRECTION('axis',(0.,0.,1.));
#22777=DIRECTION('refdir',(1.,0.,0.));
#22778=DIRECTION('center_axis',(-1.,0.,0.));
#22779=DIRECTION('ref_axis',(0.,0.,-1.));
#22780=DIRECTION('center_axis',(-1.,0.,0.));
#22781=DIRECTION('ref_axis',(0.,0.,-1.));
#22782=DIRECTION('',(0.707106781186547,-8.65956056235494E-17,-0.707106781186548));
#22783=DIRECTION('center_axis',(1.,0.,0.));
#22784=DIRECTION('ref_axis',(0.,0.,-1.));
#22785=DIRECTION('center_axis',(1.,0.,0.));
#22786=DIRECTION('ref_axis',(0.,0.,-1.));
#22787=DIRECTION('',(1.,0.,0.));
#22788=DIRECTION('center_axis',(-1.,0.,0.));
#22789=DIRECTION('ref_axis',(0.,0.,-1.));
#22790=DIRECTION('center_axis',(1.,0.,0.));
#22791=DIRECTION('ref_axis',(0.,0.,-1.));
#22792=DIRECTION('center_axis',(-1.,0.,0.));
#22793=DIRECTION('ref_axis',(0.,1.,0.));
#22794=DIRECTION('center_axis',(1.,0.,0.));
#22795=DIRECTION('ref_axis',(0.,0.,-1.));
#22796=DIRECTION('center_axis',(1.,0.,0.));
#22797=DIRECTION('ref_axis',(0.,0.,-1.));
#22798=DIRECTION('',(-0.707106781186547,8.65956056235493E-17,-0.707106781186547));
#22799=DIRECTION('center_axis',(1.,0.,0.));
#22800=DIRECTION('ref_axis',(0.,0.,-1.));
#22801=DIRECTION('center_axis',(-1.,0.,0.));
#22802=DIRECTION('ref_axis',(0.,1.,0.));
#22803=DIRECTION('center_axis',(-1.,0.,-2.85780237930534E-15));
#22804=DIRECTION('ref_axis',(0.,1.,3.18764105070188E-17));
#22805=DIRECTION('',(-0.261545900451064,-0.965191039099122,-8.96415134046473E-16));
#22806=DIRECTION('center_axis',(1.,0.,0.));
#22807=DIRECTION('ref_axis',(0.,1.,6.12323399573677E-17));
#22808=DIRECTION('center_axis',(1.,0.,0.));
#22809=DIRECTION('ref_axis',(0.,1.,6.12323399573677E-17));
#22810=DIRECTION('center_axis',(1.,0.,0.));
#22811=DIRECTION('ref_axis',(0.,1.,6.12323399573677E-17));
#22812=DIRECTION('center_axis',(1.,0.,0.));
#22813=DIRECTION('ref_axis',(0.,1.,6.12323399573677E-17));
#22814=DIRECTION('center_axis',(1.,0.,0.));
#22815=DIRECTION('ref_axis',(0.,1.,6.12323399573677E-17));
#22816=DIRECTION('center_axis',(1.,0.,0.));
#22817=DIRECTION('ref_axis',(0.,1.,6.12323399573677E-17));
#22818=DIRECTION('center_axis',(-1.,0.,0.));
#22819=DIRECTION('ref_axis',(0.,1.,0.));
#22820=DIRECTION('center_axis',(-1.,0.,0.));
#22821=DIRECTION('ref_axis',(0.,1.,0.));
#22822=DIRECTION('center_axis',(-1.,0.,0.));
#22823=DIRECTION('ref_axis',(0.,1.,0.));
#22824=DIRECTION('center_axis',(-1.,0.,0.));
#22825=DIRECTION('ref_axis',(0.,1.,0.));
#22826=DIRECTION('center_axis',(-1.,0.,0.));
#22827=DIRECTION('ref_axis',(0.,1.,0.));
#22828=DIRECTION('center_axis',(-1.,0.,0.));
#22829=DIRECTION('ref_axis',(0.,1.,0.));
#22830=DIRECTION('center_axis',(0.367220154484801,0.805519719562706,-0.46506702692814));
#22831=DIRECTION('ref_axis',(-0.784831896934838,0.,-0.61970871669976));
#22832=DIRECTION('',(0.,-0.499999999999997,-0.86602540378444));
#22833=DIRECTION('center_axis',(0.3672201544848,-9.20177782101458E-13,-0.93013405385469));
#22834=DIRECTION('ref_axis',(-0.93013405385469,0.,-0.3672201544848));
#22835=DIRECTION('',(-3.05232172441836E-15,-1.,0.));
#22836=DIRECTION('center_axis',(0.367220154484803,0.805519719563624,0.465067026926548));
#22837=DIRECTION('ref_axis',(0.784831896933805,0.,-0.619708716701069));
#22838=DIRECTION('',(0.,0.499999999999999,-0.866025403784439));
#22839=DIRECTION('center_axis',(0.367220154484804,-0.805519719563622,-0.46506702692655));
#22840=DIRECTION('ref_axis',(-0.784831896933805,0.,-0.619708716701069));
#22841=DIRECTION('',(9.15696517325506E-15,-0.499999999999999,0.866025403784439));
#22842=DIRECTION('center_axis',(0.3672201544848,9.17903343076173E-13,0.93013405385469));
#22843=DIRECTION('ref_axis',(0.93013405385469,0.,-0.3672201544848));
#22844=DIRECTION('',(-1.52616086220918E-15,1.,3.05232172441836E-15));
#22845=DIRECTION('center_axis',(0.367220154484798,-0.805519719562705,0.465067026928142));
#22846=DIRECTION('ref_axis',(0.784831896934842,0.,-0.619708716699756));
#22847=DIRECTION('',(-3.05232172441835E-15,0.499999999999999,0.866025403784439));
#22848=DIRECTION('center_axis',(0.,-0.866025403784439,0.499999999999999));
#22849=DIRECTION('ref_axis',(0.,-0.499999999999999,-0.866025403784439));
#22850=DIRECTION('',(1.,0.,0.));
#22851=DIRECTION('',(-1.,0.,0.));
#22852=DIRECTION('center_axis',(0.,-3.05232172441836E-15,1.));
#22853=DIRECTION('ref_axis',(1.,0.,0.));
#22854=DIRECTION('',(1.,0.,0.));
#22855=DIRECTION('',(-1.,0.,0.));
#22856=DIRECTION('center_axis',(0.,-0.866025403784439,-0.499999999999999));
#22857=DIRECTION('ref_axis',(0.,0.499999999999999,-0.866025403784439));
#22858=DIRECTION('',(1.,0.,0.));
#22859=DIRECTION('',(-1.,0.,0.));
#22860=DIRECTION('center_axis',(0.,0.866025403784439,0.499999999999999));
#22861=DIRECTION('ref_axis',(0.,-0.499999999999999,0.866025403784439));
#22862=DIRECTION('',(1.,0.,0.));
#22863=DIRECTION('',(-1.,0.,0.));
#22864=DIRECTION('center_axis',(0.,0.,-1.));
#22865=DIRECTION('ref_axis',(-1.,0.,0.));
#22866=DIRECTION('',(1.,0.,0.));
#22867=DIRECTION('',(-1.,0.,0.));
#22868=DIRECTION('center_axis',(0.,0.86602540378444,-0.499999999999997));
#22869=DIRECTION('ref_axis',(0.,0.499999999999997,0.86602540378444));
#22870=DIRECTION('',(1.,0.,0.));
#22871=DIRECTION('',(-1.,0.,0.));
#22872=DIRECTION('center_axis',(0.,0.5,0.866025403784439));
#22873=DIRECTION('ref_axis',(0.,-0.866025403784439,0.5));
#22874=DIRECTION('center_axis',(0.,1.,-3.84592537276713E-16));
#22875=DIRECTION('ref_axis',(0.,3.84592537276713E-16,1.));
#22876=DIRECTION('center_axis',(0.,0.5,-0.866025403784439));
#22877=DIRECTION('ref_axis',(0.,0.866025403784439,0.5));
#22878=DIRECTION('center_axis',(1.,0.,0.));
#22879=DIRECTION('ref_axis',(0.,1.,0.));
#22880=DIRECTION('',(0.504883518856957,-0.863187483914483,-1.05709978923993E-16));
#22881=DIRECTION('center_axis',(0.,-0.5,-0.866025403784439));
#22882=DIRECTION('ref_axis',(0.,0.866025403784439,-0.5));
#22883=DIRECTION('center_axis',(0.,-1.,-1.92296268638356E-16));
#22884=DIRECTION('ref_axis',(0.,1.92296268638356E-16,-1.));
#22885=DIRECTION('center_axis',(0.,-0.5,0.866025403784439));
#22886=DIRECTION('ref_axis',(0.,-0.866025403784439,-0.5));
#33205=CARTESIAN_POINT('',(0.,0.,0.));
#33206=CARTESIAN_POINT('Origin',(0.105,0.,0.));
#33207=CARTESIAN_POINT('',(0.,3.99234856522037E-16,3.26));
#33208=CARTESIAN_POINT('Origin',(0.,0.,0.));
#33209=CARTESIAN_POINT('',(0.21,-3.73517273739943E-16,3.05));
#33210=CARTESIAN_POINT('',(0.105,3.8637606513099E-16,3.155));
#33211=CARTESIAN_POINT('Origin',(0.21,0.,0.));
#33212=CARTESIAN_POINT('Origin',(0.,0.,0.));
#33213=CARTESIAN_POINT('',(4.99,3.73517273739943E-16,3.05));
#33214=CARTESIAN_POINT('',(0.,-3.73517273739943E-16,3.05));
#33215=CARTESIAN_POINT('Origin',(4.99,0.,0.));
#33216=CARTESIAN_POINT('Origin',(0.,0.,0.));
#33217=CARTESIAN_POINT('',(0.,-4.76709676493043,5.83800979439775E-16));
#33218=CARTESIAN_POINT('Origin',(0.,0.,0.));
#33219=CARTESIAN_POINT('Origin',(5.095,0.,0.));
#33220=CARTESIAN_POINT('',(5.2,-3.99234856522037E-16,3.26));
#33221=CARTESIAN_POINT('Origin',(5.2,0.,0.));
#33222=CARTESIAN_POINT('',(5.095,-3.8637606513099E-16,3.155));
#33223=CARTESIAN_POINT('Origin',(5.2,0.,0.));
#33224=CARTESIAN_POINT('',(5.2,-4.55709676493043,5.58083396657681E-16));
#33225=CARTESIAN_POINT('Origin',(5.2,0.,0.));
#33226=CARTESIAN_POINT('Origin',(5.14698723052002,0.,-1.51500018753453E-16));
#33227=CARTESIAN_POINT('',(5.12242284024924,-4.84634925793137,0.000544850078605702));
#33228=CARTESIAN_POINT('',(5.14698723052002,-4.75273145074145,-8.85041773342654E-16));
#33229=CARTESIAN_POINT('',(5.09683111434416,-4.81710063273169,-1.12843168478692));
#33230=CARTESIAN_POINT('Ctrl Pts',(5.12242284024924,-4.84634925793137,0.000544850078605714));
#33231=CARTESIAN_POINT('Ctrl Pts',(5.12258745506561,-4.84634360853001,-0.0466128059954816));
#33232=CARTESIAN_POINT('Ctrl Pts',(5.12261509827417,-4.84618263351447,-0.0937728862634767));
#33233=CARTESIAN_POINT('Ctrl Pts',(5.12249850969393,-4.84586645506482,-0.140950755812712));
#33234=CARTESIAN_POINT('Ctrl Pts',(5.1222390372062,-4.84516278744378,-0.245946966870691));
#33235=CARTESIAN_POINT('Ctrl Pts',(5.12126403884311,-4.84369122988508,-0.350884456461739));
#33236=CARTESIAN_POINT('Ctrl Pts',(5.1195137951287,-4.84146093806515,-0.455914997135786));
#33237=CARTESIAN_POINT('Ctrl Pts',(5.11919231896539,-4.84105128902516,-0.475206490639806));
#33238=CARTESIAN_POINT('Ctrl Pts',(5.11884478359864,-4.84061603078406,-0.494501019604373));
#33239=CARTESIAN_POINT('Ctrl Pts',(5.11847095209106,-4.84015520444964,-0.5137993676135));
#33240=CARTESIAN_POINT('Ctrl Pts',(5.11663697723163,-4.83789444286382,-0.60847486809847));
#33241=CARTESIAN_POINT('Ctrl Pts',(5.11417276747822,-4.83502173710584,-0.703081226948676));
#33242=CARTESIAN_POINT('Ctrl Pts',(5.11105950361714,-4.83155152799433,-0.797731355339415));
#33243=CARTESIAN_POINT('Ctrl Pts',(5.10808469285799,-4.82823564605754,-0.888172202262667));
#33244=CARTESIAN_POINT('Ctrl Pts',(5.10451721810229,-4.82437416311071,-0.978653212545341));
#33245=CARTESIAN_POINT('Ctrl Pts',(5.10036110005478,-4.81997832709177,-1.06922898060177));
#33246=CARTESIAN_POINT('Ctrl Pts',(5.09946985787141,-4.81903567954267,-1.08865214047379));
#33247=CARTESIAN_POINT('Ctrl Pts',(5.09855162625204,-4.81806845645995,-1.10807948523719));
#33248=CARTESIAN_POINT('Ctrl Pts',(5.097606577682,-4.81707676405073,-1.12751126351893));
#33249=CARTESIAN_POINT('',(5.09677740552866,-3.38580646785427,-3.60751378519044));
#33250=CARTESIAN_POINT('Origin',(5.09397446104004,0.,-3.03000037506907E-16));
#33251=CARTESIAN_POINT('',(5.09429707896,-1.43134944939545,-4.73604420895221));
#33252=CARTESIAN_POINT('Ctrl Pts',(5.09755445426771,-3.38498180226697,-3.60796213827666));
#33253=CARTESIAN_POINT('Ctrl Pts',(5.10208910805487,-3.306532374156,-3.65875518959754));
#33254=CARTESIAN_POINT('Ctrl Pts',(5.10600293671798,-3.22788838889819,-3.70900942659254));
#33255=CARTESIAN_POINT('Ctrl Pts',(5.10928749257359,-3.14899825590931,-3.75874007608228));
#33256=CARTESIAN_POINT('Ctrl Pts',(5.1125720484292,-3.07010812292044,-3.80847072557203));
#33257=CARTESIAN_POINT('Ctrl Pts',(5.1152275551448,-2.99097139609486,-3.8576781071415));
#33258=CARTESIAN_POINT('Ctrl Pts',(5.1172683027408,-2.91149242928002,-3.90640134624237));
#33259=CARTESIAN_POINT('Ctrl Pts',(5.1195258017243,-2.82357186176538,-3.96029956616864));
#33260=CARTESIAN_POINT('Ctrl Pts',(5.12102533344247,-2.73538901539391,-4.01351009532352));
#33261=CARTESIAN_POINT('Ctrl Pts',(5.12181201357767,-2.6468245785265,-4.06609184584734));
#33262=CARTESIAN_POINT('Ctrl Pts',(5.12201372622946,-2.62411577145884,-4.07957433238664));
#33263=CARTESIAN_POINT('Ctrl Pts',(5.12216874303548,-2.60138168140064,-4.09301556871597));
#33264=CARTESIAN_POINT('Ctrl Pts',(5.12227816274004,-2.57861993944308,-4.10641670396003));
#33265=CARTESIAN_POINT('Ctrl Pts',(5.12272295365878,-2.48609349589572,-4.1608922966428));
#33266=CARTESIAN_POINT('Ctrl Pts',(5.1224108220235,-2.39324441111108,-4.2146269541486));
#33267=CARTESIAN_POINT('Ctrl Pts',(5.12143116018516,-2.29992768622846,-4.26770105548192));
#33268=CARTESIAN_POINT('Ctrl Pts',(5.1207402031598,-2.23411125435542,-4.30513430208397));
#33269=CARTESIAN_POINT('Ctrl Pts',(5.11971882252206,-2.16812718645086,-4.34220177245049));
#33270=CARTESIAN_POINT('Ctrl Pts',(5.11840412361931,-2.10192539895917,-4.37893444709976));
#33271=CARTESIAN_POINT('Ctrl Pts',(5.11756105808869,-2.05947275449227,-4.40248968988531));
#33272=CARTESIAN_POINT('Ctrl Pts',(5.11659741488945,-2.01693068142318,-4.42590716144565));
#33273=CARTESIAN_POINT('Ctrl Pts',(5.1155040557362,-1.97428781828196,-4.44919441992967));
#33274=CARTESIAN_POINT('Ctrl Pts',(5.11337841852356,-1.89138435835654,-4.49446798174724));
#33275=CARTESIAN_POINT('Ctrl Pts',(5.11076604974616,-1.80824095512528,-4.53917184750963));
#33276=CARTESIAN_POINT('Ctrl Pts',(5.1076105966465,-1.72476531763046,-4.58337685908149));
#33277=CARTESIAN_POINT('Ctrl Pts',(5.10460439266534,-1.64523797691552,-4.62549102702422));
#33278=CARTESIAN_POINT('Ctrl Pts',(5.10110512412939,-1.5654088999758,-4.66715243744714));
#33279=CARTESIAN_POINT('Ctrl Pts',(5.09708531259065,-1.48523497413254,-4.7083994075618));
#33280=CARTESIAN_POINT('Ctrl Pts',(5.09618881912773,-1.46735468304869,-4.71759825649204));
#33281=CARTESIAN_POINT('Ctrl Pts',(5.09526652679194,-1.44945739634337,-4.72677639755234));
#33282=CARTESIAN_POINT('Ctrl Pts',(5.09431829354256,-1.43154291244923,-4.73593408953816));
#33283=CARTESIAN_POINT('',(5.09677740552865,1.43129534855037,-4.73595130605467));
#33284=CARTESIAN_POINT('Origin',(5.09397446104004,0.,-3.03000037506907E-16));
#33285=CARTESIAN_POINT('',(5.09429707895991,3.38585987370109,-3.60760708934543));
#33286=CARTESIAN_POINT('Ctrl Pts',(5.09755445426772,1.43209596650657,-4.73546130124953));
#33287=CARTESIAN_POINT('Ctrl Pts',(5.10208910805488,1.51530875334164,-4.69291862925353));
#33288=CARTESIAN_POINT('Ctrl Pts',(5.10600293671799,1.59815219185601,-4.64993805866292));
#33289=CARTESIAN_POINT('Ctrl Pts',(5.1092874925736,1.68066526415526,-4.60648252413149));
#33290=CARTESIAN_POINT('Ctrl Pts',(5.1125720484292,1.76317833645451,-4.56302698960007));
#33291=CARTESIAN_POINT('Ctrl Pts',(5.1152275551448,1.84536154236019,-4.5190962645815));
#33292=CARTESIAN_POINT('Ctrl Pts',(5.1172683027408,1.92729658858363,-4.47462707980373));
#33293=CARTESIAN_POINT('Ctrl Pts',(5.11952580172424,2.01793410001322,-4.42543474478548));
#33294=CARTESIAN_POINT('Ctrl Pts',(5.12102533344239,2.10810719319333,-4.37567142422865));
#33295=CARTESIAN_POINT('Ctrl Pts',(5.12181201357761,2.19792654335358,-4.325263247293));
#33296=CARTESIAN_POINT('Ctrl Pts',(5.12201372622942,2.22095712273921,-4.31233808675098));
#33297=CARTESIAN_POINT('Ctrl Pts',(5.12216874303546,2.24396461989036,-4.29937040539186));
#33298=CARTESIAN_POINT('Ctrl Pts',(5.12227816274004,2.26695121443263,-4.2863587262428));
#33299=CARTESIAN_POINT('Ctrl Pts',(5.12272295365878,2.36039168335589,-4.23346627195029));
#33300=CARTESIAN_POINT('Ctrl Pts',(5.1224108220235,2.45335180421185,-4.17992393456159));
#33301=CARTESIAN_POINT('Ctrl Pts',(5.12143116018516,2.5459736866908,-4.12564633088196));
#33302=CARTESIAN_POINT('Ctrl Pts',(5.12074020315979,2.61130004513081,-4.08736425219449));
#33303=CARTESIAN_POINT('Ctrl Pts',(5.11971882252206,2.6763934500745,-4.04875410832737));
#33304=CARTESIAN_POINT('Ctrl Pts',(5.11840412361931,2.74130577321557,-4.00978801590827));
#33305=CARTESIAN_POINT('Ctrl Pts',(5.1175610580887,2.78293153409362,-3.98480056873488));
#33306=CARTESIAN_POINT('Ctrl Pts',(5.11659741488945,2.82448269589182,-3.95966678850756));
#33307=CARTESIAN_POINT('Ctrl Pts',(5.1155040557362,2.8659714848941,-3.93438061497915));
#33308=CARTESIAN_POINT('Ctrl Pts',(5.11337841852354,2.94663126951159,-3.88522089353032));
#33309=CARTESIAN_POINT('Ctrl Pts',(5.1107660497461,3.02691765452577,-3.83556852705556));
#33310=CARTESIAN_POINT('Ctrl Pts',(5.10761059664638,3.10693813626994,-3.78537901017327));
#33311=CARTESIAN_POINT('Ctrl Pts',(5.10460439266523,3.18317374592452,-3.7375633967904));
#33312=CARTESIAN_POINT('Ctrl Pts',(5.1011051241293,3.25916812417756,-3.68926009341173));
#33313=CARTESIAN_POINT('Ctrl Pts',(5.09708531259058,3.33497601104708,-3.64045092196801));
#33314=CARTESIAN_POINT('Ctrl Pts',(5.09618881912768,3.35188259344778,-3.62956556012772));
#33315=CARTESIAN_POINT('Ctrl Pts',(5.09526652679191,3.36877974011778,-3.6186551257125));
#33316=CARTESIAN_POINT('Ctrl Pts',(5.09431829354256,3.3856677759642,-3.60771957355765));
#33317=CARTESIAN_POINT('',(5.09683109738054,4.81710063325383,-1.12843170492155));
#33318=CARTESIAN_POINT('Origin',(5.09397446104004,0.,-3.03000037506907E-16));
#33319=CARTESIAN_POINT('',(5.09435863143588,4.81720827487948,1.128405867392));
#33320=CARTESIAN_POINT('Ctrl Pts',(5.097606577682,4.81707676405073,-1.12751126351891));
#33321=CARTESIAN_POINT('Ctrl Pts',(5.10214583424673,4.82184006026792,-1.03417656102222));
#33322=CARTESIAN_POINT('Ctrl Pts',(5.10606427104759,4.82603945478669,-0.940942768451708));
#33323=CARTESIAN_POINT('Ctrl Pts',(5.10935323920574,4.82966233995838,-0.847757552481685));
#33324=CARTESIAN_POINT('Ctrl Pts',(5.11264220736389,4.83328522513008,-0.754572336511663));
#33325=CARTESIAN_POINT('Ctrl Pts',(5.11530193004546,4.83633165463593,-0.661435150975137));
#33326=CARTESIAN_POINT('Ctrl Pts',(5.11734647648754,4.83878768962393,-0.568243556567847));
#33327=CARTESIAN_POINT('Ctrl Pts',(5.11960814356782,4.84150454328205,-0.465155479480455));
#33328=CARTESIAN_POINT('Ctrl Pts',(5.12111134706416,4.84349472815332,-0.362183990119648));
#33329=CARTESIAN_POINT('Ctrl Pts',(5.12190089378603,4.84474960957374,-0.259196249019833));
#33330=CARTESIAN_POINT('Ctrl Pts',(5.12210335647361,4.84507139757935,-0.232787204091984));
#33331=CARTESIAN_POINT('Ctrl Pts',(5.12225906344213,4.84534481516978,-0.206376876932988));
#33332=CARTESIAN_POINT('Ctrl Pts',(5.12236910852286,4.84556967306519,-0.179962639911952));
#33333=CARTESIAN_POINT('Ctrl Pts',(5.12281641519127,4.84648366608875,-0.0725951475894643));
#33334=CARTESIAN_POINT('Ctrl Pts',(5.12250581136907,4.846594678656,0.0346815034442518));
#33335=CARTESIAN_POINT('Ctrl Pts',(5.12152637326862,4.84589982554879,0.142033144882093));
#33336=CARTESIAN_POINT('Ctrl Pts',(5.12083557404595,4.84540974456652,0.217748425331946));
#33337=CARTESIAN_POINT('Ctrl Pts',(5.1198137027769,4.8445190804778,0.293426134197082));
#33338=CARTESIAN_POINT('Ctrl Pts',(5.11849777244951,4.84322962374661,0.369125157802716));
#33339=CARTESIAN_POINT('Ctrl Pts',(5.11765391725392,4.8424027450438,0.417668012269155));
#33340=CARTESIAN_POINT('Ctrl Pts',(5.11668918025442,4.84141184227801,0.466219495085933));
#33341=CARTESIAN_POINT('Ctrl Pts',(5.1155944719316,4.84025777988173,0.514793214344727));
#33342=CARTESIAN_POINT('Ctrl Pts',(5.1134660840762,4.83801399280399,0.609232721205176));
#33343=CARTESIAN_POINT('Ctrl Pts',(5.11084994672088,4.83515680140141,0.703595379434204));
#33344=CARTESIAN_POINT('Ctrl Pts',(5.10769005829827,4.83170141167255,0.797996480817579));
#33345=CARTESIAN_POINT('Ctrl Pts',(5.10467957854565,4.82840940277069,0.887934024911113));
#33346=CARTESIAN_POINT('Ctrl Pts',(5.10117541306817,4.8245743529801,0.977906636196995));
#33347=CARTESIAN_POINT('Ctrl Pts',(5.09715037047566,4.82020789063866,1.06797075806217));
#33348=CARTESIAN_POINT('Ctrl Pts',(5.0962533412586,4.81923477191869,1.08804263230067));
#33349=CARTESIAN_POINT('Ctrl Pts',(5.0953305327574,4.81823525539394,1.10811886917062));
#33350=CARTESIAN_POINT('Ctrl Pts',(5.09438180624853,4.81720946415242,1.12819977138991));
#33351=CARTESIAN_POINT('',(5.09677740552871,3.38580646785444,3.60751378519034));
#33352=CARTESIAN_POINT('Origin',(5.09397446104004,0.,-3.03000037506907E-16));
#33353=CARTESIAN_POINT('',(5.09429707895988,1.43134944939528,4.73604420895232));
#33354=CARTESIAN_POINT('Ctrl Pts',(5.09755445426767,3.38498180226722,3.60796213827651));
#33355=CARTESIAN_POINT('Ctrl Pts',(5.10208910805484,3.3065323741562,3.65875518959743));
#33356=CARTESIAN_POINT('Ctrl Pts',(5.10600293671795,3.22788838889833,3.70900942659247));
#33357=CARTESIAN_POINT('Ctrl Pts',(5.10928749257356,3.14899825590938,3.75874007608226));
#33358=CARTESIAN_POINT('Ctrl Pts',(5.11257204842918,3.07010812292043,3.80847072557205));
#33359=CARTESIAN_POINT('Ctrl Pts',(5.11522755514478,2.99097139609477,3.85767810714158));
#33360=CARTESIAN_POINT('Ctrl Pts',(5.11726830274078,2.91149242927984,3.90640134624249));
#33361=CARTESIAN_POINT('Ctrl Pts',(5.11952580172432,2.82357186176373,3.96029956616967));
#33362=CARTESIAN_POINT('Ctrl Pts',(5.1210253334425,2.73538901539079,4.01351009532541));
#33363=CARTESIAN_POINT('Ctrl Pts',(5.12181201357769,2.64682457852191,4.06609184585008));
#33364=CARTESIAN_POINT('Ctrl Pts',(5.12201372622945,2.62411577145574,4.07957433238849));
#33365=CARTESIAN_POINT('Ctrl Pts',(5.12216874303546,2.60138168139903,4.09301556871694));
#33366=CARTESIAN_POINT('Ctrl Pts',(5.12227816274002,2.57861993944296,4.10641670396012));
#33367=CARTESIAN_POINT('Ctrl Pts',(5.12272295365876,2.48609349589551,4.16089229664294));
#33368=CARTESIAN_POINT('Ctrl Pts',(5.12241082202347,2.39324441111092,4.21462695414871));
#33369=CARTESIAN_POINT('Ctrl Pts',(5.12143116018513,2.29992768622834,4.26770105548201));
#33370=CARTESIAN_POINT('Ctrl Pts',(5.12074020315977,2.23411125435535,4.30513430208403));
#33371=CARTESIAN_POINT('Ctrl Pts',(5.11971882252203,2.16812718645086,4.34220177245051));
#33372=CARTESIAN_POINT('Ctrl Pts',(5.11840412361928,2.10192539895918,4.37893444709977));
#33373=CARTESIAN_POINT('Ctrl Pts',(5.11756105808867,2.05947275449225,4.40248968988534));
#33374=CARTESIAN_POINT('Ctrl Pts',(5.11659741488942,2.0169306814231,4.42590716144571));
#33375=CARTESIAN_POINT('Ctrl Pts',(5.11550405573616,1.97428781828179,4.44919441992978));
#33376=CARTESIAN_POINT('Ctrl Pts',(5.11337841852356,1.8913843583577,4.49446798174663));
#33377=CARTESIAN_POINT('Ctrl Pts',(5.11076604974621,1.80824095512778,4.53917184750831));
#33378=CARTESIAN_POINT('Ctrl Pts',(5.10761059664661,1.72476531763432,4.58337685907947));
#33379=CARTESIAN_POINT('Ctrl Pts',(5.10460439266551,1.64523797692054,4.62549102702161));
#33380=CARTESIAN_POINT('Ctrl Pts',(5.10110512412964,1.565408899982,4.66715243744393));
#33381=CARTESIAN_POINT('Ctrl Pts',(5.09708531259098,1.48523497413995,4.70839940755801));
#33382=CARTESIAN_POINT('Ctrl Pts',(5.09618881912794,1.46735468305352,4.71759825648959));
#33383=CARTESIAN_POINT('Ctrl Pts',(5.09526652679202,1.44945739634561,4.72677639755122));
#33384=CARTESIAN_POINT('Ctrl Pts',(5.09431829354251,1.43154291244888,4.73593408953836));
#33385=CARTESIAN_POINT('',(5.09677740552872,-1.43129534855014,4.73595130605479));
#33386=CARTESIAN_POINT('Origin',(5.09397446104004,0.,-3.03000037506907E-16));
#33387=CARTESIAN_POINT('',(5.09429707895997,-3.38585987370121,3.60760708934535));
#33388=CARTESIAN_POINT('Ctrl Pts',(5.09755445426766,-1.43209596650623,4.73546130124972));
#33389=CARTESIAN_POINT('Ctrl Pts',(5.10208910805483,-1.51530875334136,4.69291862925369));
#33390=CARTESIAN_POINT('Ctrl Pts',(5.10600293671795,-1.5981521918558,4.64993805866305));
#33391=CARTESIAN_POINT('Ctrl Pts',(5.10928749257356,-1.68066526415513,4.60648252413158));
#33392=CARTESIAN_POINT('Ctrl Pts',(5.11257204842917,-1.76317833645446,4.56302698960011));
#33393=CARTESIAN_POINT('Ctrl Pts',(5.11522755514477,-1.84536154236023,4.5190962645815));
#33394=CARTESIAN_POINT('Ctrl Pts',(5.11726830274077,-1.92729658858375,4.47462707980369));
#33395=CARTESIAN_POINT('Ctrl Pts',(5.11952580172431,-2.01793410001716,4.42543474478336));
#33396=CARTESIAN_POINT('Ctrl Pts',(5.12102533344249,-2.10810719320099,4.37567142422444));
#33397=CARTESIAN_POINT('Ctrl Pts',(5.12181201357768,-2.19792654336493,4.32526324728665));
#33398=CARTESIAN_POINT('Ctrl Pts',(5.12201372622944,-2.22095712274679,4.31233808674672));
#33399=CARTESIAN_POINT('Ctrl Pts',(5.12216874303545,-2.24396461989418,4.29937040538972));
#33400=CARTESIAN_POINT('Ctrl Pts',(5.12227816274001,-2.2669512144327,4.28635872624278));
#33401=CARTESIAN_POINT('Ctrl Pts',(5.12272295365876,-2.36039168335588,4.23346627195032));
#33402=CARTESIAN_POINT('Ctrl Pts',(5.12241082202347,-2.45335180421187,4.17992393456159));
#33403=CARTESIAN_POINT('Ctrl Pts',(5.12143116018513,-2.54597368669086,4.12564633088194));
#33404=CARTESIAN_POINT('Ctrl Pts',(5.12074020315977,-2.61130004513086,4.08736425219448));
#33405=CARTESIAN_POINT('Ctrl Pts',(5.11971882252203,-2.67639345007453,4.04875410832738));
#33406=CARTESIAN_POINT('Ctrl Pts',(5.11840412361928,-2.74130577321558,4.00978801590828));
#33407=CARTESIAN_POINT('Ctrl Pts',(5.11756105808867,-2.78293153409365,3.98480056873488));
#33408=CARTESIAN_POINT('Ctrl Pts',(5.11659741488943,-2.82448269589188,3.95966678850754));
#33409=CARTESIAN_POINT('Ctrl Pts',(5.11550405573617,-2.86597148489419,3.93438061497911));
#33410=CARTESIAN_POINT('Ctrl Pts',(5.11337841852351,-2.94663126951153,3.88522089353037));
#33411=CARTESIAN_POINT('Ctrl Pts',(5.11076604974608,-3.02691765452555,3.83556852705571));
#33412=CARTESIAN_POINT('Ctrl Pts',(5.10761059664637,-3.10693813626956,3.78537901017352));
#33413=CARTESIAN_POINT('Ctrl Pts',(5.10460439266523,-3.18317374592392,3.73756339679079));
#33414=CARTESIAN_POINT('Ctrl Pts',(5.10110512412932,-3.25916812417675,3.68926009341227));
#33415=CARTESIAN_POINT('Ctrl Pts',(5.09708531259061,-3.33497601104604,3.64045092196869));
#33416=CARTESIAN_POINT('Ctrl Pts',(5.09618881912769,-3.35188259344717,3.62956556012812));
#33417=CARTESIAN_POINT('Ctrl Pts',(5.0952665267919,-3.3687797401176,3.61865512571262));
#33418=CARTESIAN_POINT('Ctrl Pts',(5.09431829354252,-3.38566777596445,3.6077195735575));
#33419=CARTESIAN_POINT('',(5.09422149081015,-4.81720123716838,1.12962547313837));
#33420=CARTESIAN_POINT('Origin',(5.09397446104004,0.,-3.03000037506907E-16));
#33421=CARTESIAN_POINT('Ctrl Pts',(5.09438180624853,-4.81720946415242,1.12819977138992));
#33422=CARTESIAN_POINT('Ctrl Pts',(5.09878886055567,-4.82197450198674,1.03491933093676));
#33423=CARTESIAN_POINT('Ctrl Pts',(5.10263430365562,-4.82617320749278,0.941738192636836));
#33424=CARTESIAN_POINT('Ctrl Pts',(5.10594351391264,-4.82979238468145,0.848601343867398));
#33425=CARTESIAN_POINT('Ctrl Pts',(5.10925272416967,-4.83341156187012,0.75546449509796));
#33426=CARTESIAN_POINT('Ctrl Pts',(5.11202603583231,-4.8364512781726,0.662371388440315));
#33427=CARTESIAN_POINT('Ctrl Pts',(5.11431327464526,-4.83889682851293,0.569216691291326));
#33428=CARTESIAN_POINT('Ctrl Pts',(5.11595169894918,-4.84064865656489,0.502486921330922));
#33429=CARTESIAN_POINT('Ctrl Pts',(5.11733887369218,-4.84209375534294,0.435801442391284));
#33430=CARTESIAN_POINT('Ctrl Pts',(5.11849784929899,-4.84322957955454,0.369125161058667));
#33431=CARTESIAN_POINT('Ctrl Pts',(5.11958756105594,-4.84429752351292,0.306433653790524));
#33432=CARTESIAN_POINT('Ctrl Pts',(5.12047576221681,-4.84509205804993,0.243750068965635));
#33433=CARTESIAN_POINT('Ctrl Pts',(5.12114133368399,-4.8456119029517,0.181040444019433));
#33434=CARTESIAN_POINT('Ctrl Pts',(5.12178006274419,-4.8461107825791,0.120859889739829));
#33435=CARTESIAN_POINT('Ctrl Pts',(5.12221296107479,-4.84635639410279,0.0607049047250273));
#33436=CARTESIAN_POINT('Ctrl Pts',(5.12242284024924,-4.84634925793137,0.000544850078605714));
#33437=CARTESIAN_POINT('Ctrl Pts',(4.44772342888108,0.165392353541528,5.67801337205715));
#33438=CARTESIAN_POINT('Ctrl Pts',(4.69727026033307,0.931491616708207,5.2357057562419));
#33439=CARTESIAN_POINT('Ctrl Pts',(4.96928012765321,2.42096936008937,4.37575538014882));
#33440=CARTESIAN_POINT('Ctrl Pts',(4.78045253748373,3.81314196223624,3.57198415354091));
#33441=CARTESIAN_POINT('Ctrl Pts',(4.44772342888108,4.83460764645847,2.98224066578724));
#33442=CARTESIAN_POINT('Ctrl Pts',(4.5447241499808,0.110261569027686,5.63725117364547));
#33443=CARTESIAN_POINT('Ctrl Pts',(4.7983881862218,0.881878377310221,5.19312555764156));
#33444=CARTESIAN_POINT('Ctrl Pts',(5.07815075443906,2.389498397681,4.32537672517764));
#33445=CARTESIAN_POINT('Ctrl Pts',(4.8829428649688,3.79962864594736,3.50901750660556));
#33446=CARTESIAN_POINT('Ctrl Pts',(4.5447241499808,4.82687193937677,2.91411490666184));
#33447=CARTESIAN_POINT('Ctrl Pts',(4.64172487108053,0.0551307845138434,
5.59648897523378));
#33448=CARTESIAN_POINT('Ctrl Pts',(4.89950611211053,0.832265137912237,5.15054535904122));
#33449=CARTESIAN_POINT('Ctrl Pts',(5.18702138122492,2.35802743527264,4.27499807020645));
#33450=CARTESIAN_POINT('Ctrl Pts',(4.98543319245386,3.78611532965848,3.44605085967021));
#33451=CARTESIAN_POINT('Ctrl Pts',(4.64172487108053,4.81913623229508,2.84598914753644));
#33452=CARTESIAN_POINT('Ctrl Pts',(4.73872559218025,1.11022302462516E-15,
5.5557267768221));
#33453=CARTESIAN_POINT('Ctrl Pts',(5.00062403799926,0.782651898514251,5.10796516044089));
#33454=CARTESIAN_POINT('Ctrl Pts',(5.29589200801077,2.32655647286427,4.22461941523526));
#33455=CARTESIAN_POINT('Ctrl Pts',(5.08792351993893,3.7726020133696,3.38308421273486));
#33456=CARTESIAN_POINT('Ctrl Pts',(4.73872559218025,4.81140052521337,2.77786338841105));
#33457=CARTESIAN_POINT('',(4.73872559218025,4.81140052521337,2.77786338841105));
#33458=CARTESIAN_POINT('Ctrl Pts',(5.097554454267,3.38498180227162,3.60796213827396));
#33459=CARTESIAN_POINT('Ctrl Pts',(5.02981162260678,3.82780377487382,3.35078704750243));
#33460=CARTESIAN_POINT('Ctrl Pts',(4.91293516184791,4.29315964422862,3.0797989125881));
#33461=CARTESIAN_POINT('Ctrl Pts',(4.73872559218025,4.81140052521337,2.77786338841105));
#33462=CARTESIAN_POINT('',(4.45307482442111,4.81813466520579,2.99175134594783));
#33463=CARTESIAN_POINT('Ctrl Pts',(4.45307482442111,4.81813466520579,2.99175134594783));
#33464=CARTESIAN_POINT('Ctrl Pts',(4.50072369957731,4.81696840196052,2.95614749038523));
#33465=CARTESIAN_POINT('Ctrl Pts',(4.54835588589747,4.81582399363754,2.92051895860767));
#33466=CARTESIAN_POINT('Ctrl Pts',(4.64357232351903,4.81357928293661,2.84922335113861));
#33467=CARTESIAN_POINT('Ctrl Pts',(4.69115813327903,4.81247893359302,2.81355512622421));
#33468=CARTESIAN_POINT('Ctrl Pts',(4.73872559218025,4.81140052521337,2.77786338841105));
#33469=CARTESIAN_POINT('',(4.45307482442096,0.181865334794732,5.66850269189626));
#33470=CARTESIAN_POINT('Ctrl Pts',(4.45307670887188,4.81813292344043,2.99175235155653));
#33471=CARTESIAN_POINT('Ctrl Pts',(4.78160975160098,3.8045770857894,3.57692908726307));
#33472=CARTESIAN_POINT('Ctrl Pts',(4.96786706546316,2.42067099411741,4.37592764182305));
#33473=CARTESIAN_POINT('Ctrl Pts',(4.69893917059593,0.940653225099449,5.230416299171));
#33474=CARTESIAN_POINT('Ctrl Pts',(4.45307570990783,0.181866974811239,5.66850174503229));
#33475=CARTESIAN_POINT('',(4.73872559218025,1.5738093079395E-15,5.5557267768221));
#33476=CARTESIAN_POINT('Ctrl Pts',(4.73872559218025,2.80742846517038E-15,
5.5557267768221));
#33477=CARTESIAN_POINT('Ctrl Pts',(4.69115755784355,0.0303711148643061,
5.57450680196497));
#33478=CARTESIAN_POINT('Ctrl Pts',(4.64357117219491,0.060710895726737,5.59329407226952));
#33479=CARTESIAN_POINT('Ctrl Pts',(4.54835473372577,0.121332346083827,5.63088585282973));
#33480=CARTESIAN_POINT('Ctrl Pts',(4.50072312329429,0.151614988891,5.64969097803559));
#33481=CARTESIAN_POINT('Ctrl Pts',(4.45307482442137,0.181865334795011,5.6685026918961));
#33482=CARTESIAN_POINT('Ctrl Pts',(4.73872559218025,1.11022302462516E-15,
5.5557267768221));
#33483=CARTESIAN_POINT('Ctrl Pts',(4.91293516184791,0.520604274734674,5.2578847706982));
#33484=CARTESIAN_POINT('Ctrl Pts',(5.02725497143633,0.98767988560083,4.99065459457934));
#33485=CARTESIAN_POINT('Ctrl Pts',(5.09431829354185,1.43154291244451,4.73593408954086));
#33486=CARTESIAN_POINT('Ctrl Pts',(4.44772342888108,5.,2.69577270626991));
#33487=CARTESIAN_POINT('Ctrl Pts',(4.69727026033307,5.,1.8111574746394));
#33488=CARTESIAN_POINT('Ctrl Pts',(4.96948022596782,5.,0.0912172907134413));
#33489=CARTESIAN_POINT('Ctrl Pts',(4.78045253748373,5.,-1.51628573076257));
#33490=CARTESIAN_POINT('Ctrl Pts',(4.44772342888108,5.,-2.69577270626992));
#33491=CARTESIAN_POINT('Ctrl Pts',(4.5447241499808,4.93713350840446,2.72313626698363));
#33492=CARTESIAN_POINT('Ctrl Pts',(4.7983881862218,4.93831784661493,1.83283370102193));
#33493=CARTESIAN_POINT('Ctrl Pts',(5.07834742005573,4.94063410426251,0.0932810725788978));
#33494=CARTESIAN_POINT('Ctrl Pts',(4.8829428649688,4.93871262601842,-1.5360661790347));
#33495=CARTESIAN_POINT('Ctrl Pts',(4.5447241499808,4.93713350840446,-2.72313626698363));
#33496=CARTESIAN_POINT('Ctrl Pts',(4.64172487108053,4.87426701680892,2.75049982769734));
#33497=CARTESIAN_POINT('Ctrl Pts',(4.89950611211053,4.87663569322986,1.85450992740445));
#33498=CARTESIAN_POINT('Ctrl Pts',(5.18721461414363,4.88126820852503,0.0953448544443543));
#33499=CARTESIAN_POINT('Ctrl Pts',(4.98543319245386,4.87742525203684,-1.55584662730683));
#33500=CARTESIAN_POINT('Ctrl Pts',(4.64172487108053,4.87426701680891,-2.75049982769734));
#33501=CARTESIAN_POINT('Ctrl Pts',(4.73872559218025,4.81140052521337,2.77786338841105));
#33502=CARTESIAN_POINT('Ctrl Pts',(5.00062403799926,4.81495353984479,1.87618615378698));
#33503=CARTESIAN_POINT('Ctrl Pts',(5.29608180823153,4.82190231278754,0.0974086363098105));
#33504=CARTESIAN_POINT('Ctrl Pts',(5.08792351993893,4.81613787805526,-1.57562707557896));
#33505=CARTESIAN_POINT('Ctrl Pts',(4.73872559218025,4.81140052521337,-2.77786338841105));
#33506=CARTESIAN_POINT('',(4.73872559218025,4.81140052521337,-2.77786338841105));
#33507=CARTESIAN_POINT('Ctrl Pts',(5.0976065776813,4.81707676405072,-1.12751126352421));
#33508=CARTESIAN_POINT('Ctrl Pts',(5.02983861611708,4.8157680729232,-1.63958805258426));
#33509=CARTESIAN_POINT('Ctrl Pts',(4.91293516184791,4.81376391896329,-2.1780858581101));
#33510=CARTESIAN_POINT('Ctrl Pts',(4.73872559218025,4.81140052521337,-2.77786338841105));
#33511=CARTESIAN_POINT('',(4.45307482442111,5.,-2.67675134594873));
#33512=CARTESIAN_POINT('Ctrl Pts',(4.45307482442111,5.,-2.67675134594873));
#33513=CARTESIAN_POINT('Ctrl Pts',(4.50072369957984,4.96858302498581,-2.69354326013303));
#33514=CARTESIAN_POINT('Ctrl Pts',(4.54835588589865,4.9371556072063,-2.71036643934133));
#33515=CARTESIAN_POINT('Ctrl Pts',(4.64357232350986,4.87428944461622,-2.74407026658104));
#33516=CARTESIAN_POINT('Ctrl Pts',(4.69115813327444,4.84284968105765,-2.76095144855526));
#33517=CARTESIAN_POINT('Ctrl Pts',(4.73872559218026,4.81140052521337,-2.77786338841105));
#33518=CARTESIAN_POINT('',(4.45307482442096,5.,2.67675134594813));
#33519=CARTESIAN_POINT('Ctrl Pts',(4.45307671877181,5.,-2.67674933668223));
#33520=CARTESIAN_POINT('Ctrl Pts',(4.78161097872069,5.,-1.50639610513671));
#33521=CARTESIAN_POINT('Ctrl Pts',(4.96806593665806,5.,0.0915620558803535));
#33522=CARTESIAN_POINT('Ctrl Pts',(4.69894039771564,5.,1.80057831867916));
#33523=CARTESIAN_POINT('Ctrl Pts',(4.45307572309982,5.,2.67674944962055));
#33524=CARTESIAN_POINT('Ctrl Pts',(4.73872559218025,4.81140052521337,2.77786338841105));
#33525=CARTESIAN_POINT('Ctrl Pts',(4.69115755784416,4.84285006150256,2.76095124396896));
#33526=CARTESIAN_POINT('Ctrl Pts',(4.64357117219626,4.8742902052848,2.74406985814937));
#33527=CARTESIAN_POINT('Ctrl Pts',(4.54835473372633,4.93715636740249,2.7103660324057));
#33528=CARTESIAN_POINT('Ctrl Pts',(4.50072312329534,4.96858340495538,2.69354305704407));
#33529=CARTESIAN_POINT('Ctrl Pts',(4.45307482442137,5.,2.67675134594781));
#33530=CARTESIAN_POINT('Ctrl Pts',(4.73872559218025,4.81140052521337,2.77786338841105));
#33531=CARTESIAN_POINT('Ctrl Pts',(4.91293516184791,4.81376391896329,2.1780858581101));
#33532=CARTESIAN_POINT('Ctrl Pts',(5.02729096278339,4.81587290945609,1.63996307009543));
#33533=CARTESIAN_POINT('Ctrl Pts',(5.09438180624785,4.81720946415241,1.12819977139512));
#33534=CARTESIAN_POINT('Origin',(4.82293768228025,0.,0.));
#33535=CARTESIAN_POINT('Origin',(4.82293768228025,0.,0.));
#33536=CARTESIAN_POINT('Ctrl Pts',(4.73872559218025,4.81140052521337,-2.77786338841105));
#33537=CARTESIAN_POINT('Ctrl Pts',(4.91293516184791,4.29315964422862,-3.0797989125881));
#33538=CARTESIAN_POINT('Ctrl Pts',(5.02725497143633,3.82819371761882,-3.3506831690269));
#33539=CARTESIAN_POINT('Ctrl Pts',(5.09431829354185,3.38566777596886,-3.60771957355494));
#33540=CARTESIAN_POINT('Origin',(4.82293768228025,0.,0.));
#33541=CARTESIAN_POINT('',(4.73872559218025,-8.93429006522259E-16,-5.5557267768221));
#33542=CARTESIAN_POINT('Ctrl Pts',(4.73872559218025,2.80742846517038E-15,
-5.5557267768221));
#33543=CARTESIAN_POINT('Ctrl Pts',(4.91293516184791,-0.520604274734672,
-5.2578847706982));
#33544=CARTESIAN_POINT('Ctrl Pts',(5.02725497143632,-0.98767988560083,-4.99065459457934));
#33545=CARTESIAN_POINT('Ctrl Pts',(5.09431829354185,-1.43154291244451,-4.73593408954086));
#33546=CARTESIAN_POINT('Ctrl Pts',(5.097554454267,1.43209596650185,-4.73546130125224));
#33547=CARTESIAN_POINT('Ctrl Pts',(5.02981162260678,0.987964818372043,-4.99036883349392));
#33548=CARTESIAN_POINT('Ctrl Pts',(4.91293516184791,0.52060427473467,-5.2578847706982));
#33549=CARTESIAN_POINT('Ctrl Pts',(4.73872559218025,-3.19189119579733E-15,
-5.5557267768221));
#33550=CARTESIAN_POINT('Origin',(4.82293768228025,0.,0.));
#33551=CARTESIAN_POINT('',(4.73872559218025,-4.81140052521337,-2.77786338841105));
#33552=CARTESIAN_POINT('Ctrl Pts',(4.73872559218025,-4.81140052521337,-2.77786338841105));
#33553=CARTESIAN_POINT('Ctrl Pts',(4.91293516184791,-4.81376391896329,-2.1780858581101));
#33554=CARTESIAN_POINT('Ctrl Pts',(5.02983861611708,-4.8157680729232,-1.63958805258425));
#33555=CARTESIAN_POINT('Ctrl Pts',(5.0976065776813,-4.81707676405072,-1.12751126352421));
#33556=CARTESIAN_POINT('Ctrl Pts',(5.097554454267,-3.38498180227163,-3.60796213827395));
#33557=CARTESIAN_POINT('Ctrl Pts',(5.02981162260678,-3.82780377487383,-3.35078704750243));
#33558=CARTESIAN_POINT('Ctrl Pts',(4.91293516184791,-4.29315964422862,-3.0797989125881));
#33559=CARTESIAN_POINT('Ctrl Pts',(4.73872559218025,-4.81140052521337,-2.77786338841105));
#33560=CARTESIAN_POINT('Origin',(4.82293768228025,0.,0.));
#33561=CARTESIAN_POINT('',(4.73872559218025,-4.81140052521338,2.77786338841105));
#33562=CARTESIAN_POINT('Ctrl Pts',(4.73872559218025,-4.81140052521338,2.77786338841104));
#33563=CARTESIAN_POINT('Ctrl Pts',(4.91293516184791,-4.29315964422862,3.0797989125881));
#33564=CARTESIAN_POINT('Ctrl Pts',(5.02725497143633,-3.82819371761882,3.3506831690269));
#33565=CARTESIAN_POINT('Ctrl Pts',(5.09431829354185,-3.38566777596886,3.60771957355494));
#33566=CARTESIAN_POINT('Ctrl Pts',(5.09438180624785,-4.81720946415241,1.12819977139512));
#33567=CARTESIAN_POINT('Ctrl Pts',(5.02729096278339,-4.81587290945609,1.63996307009543));
#33568=CARTESIAN_POINT('Ctrl Pts',(4.91293516184791,-4.81376391896329,2.1780858581101));
#33569=CARTESIAN_POINT('Ctrl Pts',(4.73872559218025,-4.81140052521337,2.77786338841105));
#33570=CARTESIAN_POINT('Origin',(4.82293768228025,0.,0.));
#33571=CARTESIAN_POINT('Ctrl Pts',(5.097554454267,-1.43209596650185,4.73546130125224));
#33572=CARTESIAN_POINT('Ctrl Pts',(5.02981162260678,-0.987964818372044,
4.99036883349392));
#33573=CARTESIAN_POINT('Ctrl Pts',(4.91293516184791,-0.520604274734671,
5.2578847706982));
#33574=CARTESIAN_POINT('Ctrl Pts',(4.73872559218025,1.94289029309402E-15,
5.5557267768221));
#33575=CARTESIAN_POINT('Ctrl Pts',(4.44772342888108,4.83460764645847,-2.98224066578724));
#33576=CARTESIAN_POINT('Ctrl Pts',(4.69727026033307,4.06850838329179,-3.4245482816025));
#33577=CARTESIAN_POINT('Ctrl Pts',(4.96928012765321,2.57903063991063,-4.28449865769557));
#33578=CARTESIAN_POINT('Ctrl Pts',(4.78045253748373,1.18685803776376,-5.08826988430348));
#33579=CARTESIAN_POINT('Ctrl Pts',(4.44772342888108,0.165392353541524,-5.67801337205715));
#33580=CARTESIAN_POINT('Ctrl Pts',(4.5447241499808,4.82687193937677,-2.91411490666184));
#33581=CARTESIAN_POINT('Ctrl Pts',(4.7983881862218,4.05643946930471,-3.36029185661963));
#33582=CARTESIAN_POINT('Ctrl Pts',(5.07815075443906,2.55113692610127,-4.23205467728278));
#33583=CARTESIAN_POINT('Ctrl Pts',(4.8829428649688,1.13908398007106,-5.04508368564026));
#33584=CARTESIAN_POINT('Ctrl Pts',(4.5447241499808,0.110261569027681,-5.63725117364547));
#33585=CARTESIAN_POINT('Ctrl Pts',(4.64172487108053,4.81913623229507,-2.84598914753645));
#33586=CARTESIAN_POINT('Ctrl Pts',(4.89950611211053,4.04437055531762,-3.29603543163677));
#33587=CARTESIAN_POINT('Ctrl Pts',(5.18702138122492,2.52324321229191,-4.17961069687));
#33588=CARTESIAN_POINT('Ctrl Pts',(4.98543319245386,1.09130992237836,-5.00189748697704));
#33589=CARTESIAN_POINT('Ctrl Pts',(4.64172487108053,0.0551307845138391,
-5.59648897523378));
#33590=CARTESIAN_POINT('Ctrl Pts',(4.73872559218025,4.81140052521337,-2.77786338841105));
#33591=CARTESIAN_POINT('Ctrl Pts',(5.00062403799926,4.03230164133054,-3.23177900665391));
#33592=CARTESIAN_POINT('Ctrl Pts',(5.29589200801077,2.49534949848256,-4.12716671645721));
#33593=CARTESIAN_POINT('Ctrl Pts',(5.08792351993893,1.04353586468566,-4.95871128831382));
#33594=CARTESIAN_POINT('Ctrl Pts',(4.73872559218025,-3.19189119579733E-15,
-5.5557267768221));
#33595=CARTESIAN_POINT('',(4.45307482442111,0.181865334794207,-5.66850269189656));
#33596=CARTESIAN_POINT('Ctrl Pts',(4.45307482442111,0.181865334794213,-5.66850269189656));
#33597=CARTESIAN_POINT('Ctrl Pts',(4.50072369959053,0.151614623018565,-5.64969075051213));
#33598=CARTESIAN_POINT('Ctrl Pts',(4.54835588590384,0.121331613565481,-5.63088539794606));
#33599=CARTESIAN_POINT('Ctrl Pts',(4.64357232350899,0.0607101616799395,
-5.59329361772685));
#33600=CARTESIAN_POINT('Ctrl Pts',(4.69115813327399,0.0303707474648052,
-5.57450657478309));
#33601=CARTESIAN_POINT('Ctrl Pts',(4.73872559218025,-8.93429006522259E-16,
-5.5557267768221));
#33602=CARTESIAN_POINT('',(4.45307482442096,4.81813466520527,-2.99175134594813));
#33603=CARTESIAN_POINT('Ctrl Pts',(4.45307670887187,0.18186707655957,-5.66850168628786));
#33604=CARTESIAN_POINT('Ctrl Pts',(4.78160975160098,1.1954229142106,-5.08332495058132));
#33605=CARTESIAN_POINT('Ctrl Pts',(4.96786706546316,2.57932900588259,-4.28432639602134));
#33606=CARTESIAN_POINT('Ctrl Pts',(4.69893917059593,4.05934677490055,-3.42983773867339));
#33607=CARTESIAN_POINT('Ctrl Pts',(4.45307570990783,4.81813302518876,-2.9917522928121));
#33608=CARTESIAN_POINT('Ctrl Pts',(4.73872559218025,4.81140052521337,-2.77786338841105));
#33609=CARTESIAN_POINT('Ctrl Pts',(4.69115755784131,4.81247894663871,-2.81355555799791));
#33610=CARTESIAN_POINT('Ctrl Pts',(4.64357117219035,4.81357930955906,-2.84922421412404));
#33611=CARTESIAN_POINT('Ctrl Pts',(4.54835473372485,4.81582402131905,-2.92051982042491));
#33612=CARTESIAN_POINT('Ctrl Pts',(4.5007231232927,4.81696841606511,-2.95614792099309));
#33613=CARTESIAN_POINT('Ctrl Pts',(4.45307482442137,4.81813466520499,-2.99175134594829));
#33614=CARTESIAN_POINT('Origin',(4.45307482442111,5.,-2.67675134594873));
#33615=CARTESIAN_POINT('',(4.45307482442096,5.,-2.67675134594813));
#33616=CARTESIAN_POINT('Origin',(4.73872559218025,-8.93429006522259E-16,
-5.5557267768221));
#33617=CARTESIAN_POINT('',(4.45307482442096,-0.181865334794733,-5.66850269189626));
#33618=CARTESIAN_POINT('Ctrl Pts',(4.73872559218025,2.80742846517038E-15,
-5.5557267768221));
#33619=CARTESIAN_POINT('Ctrl Pts',(4.69115755784503,-0.0303711148633555,
-5.57450680196439));
#33620=CARTESIAN_POINT('Ctrl Pts',(4.64357117219794,-0.0607108957248108,
-5.59329407226833));
#33621=CARTESIAN_POINT('Ctrl Pts',(4.54835473372581,-0.121332346083798,
-5.63088585282971));
#33622=CARTESIAN_POINT('Ctrl Pts',(4.50072312329487,-0.151614988890633,
-5.64969097803537));
#33623=CARTESIAN_POINT('Ctrl Pts',(4.45307482442137,-0.181865334795012,
-5.6685026918961));
#33624=CARTESIAN_POINT('',(4.45307482442096,0.18186533479473,-5.66850269189626));
#33625=CARTESIAN_POINT('Origin',(4.45307482442111,4.81813466520579,2.99175134594783));
#33626=CARTESIAN_POINT('',(4.45307482442096,4.81813466520527,2.99175134594813));
#33627=CARTESIAN_POINT('Origin',(4.73872559218025,-4.81140052521337,-2.77786338841105));
#33628=CARTESIAN_POINT('',(4.45307482442111,-4.81813466520579,-2.99175134594783));
#33629=CARTESIAN_POINT('Ctrl Pts',(4.45307482442111,-4.81813466520579,-2.99175134594783));
#33630=CARTESIAN_POINT('Ctrl Pts',(4.50072369957741,-4.81696840196052,-2.95614749038515));
#33631=CARTESIAN_POINT('Ctrl Pts',(4.54835588589733,-4.81582399363755,-2.92051895860778));
#33632=CARTESIAN_POINT('Ctrl Pts',(4.64357232351839,-4.81357928293662,-2.84922335113908));
#33633=CARTESIAN_POINT('Ctrl Pts',(4.69115813327887,-4.81247893359302,-2.81355512622433));
#33634=CARTESIAN_POINT('Ctrl Pts',(4.73872559218025,-4.81140052521337,-2.77786338841105));
#33635=CARTESIAN_POINT('',(4.45307482442096,-5.,-2.67675134594813));
#33636=CARTESIAN_POINT('Ctrl Pts',(4.73872559218026,-4.81140052521337,-2.77786338841105));
#33637=CARTESIAN_POINT('Ctrl Pts',(4.69115755784151,-4.84285006150431,-2.76095124396802));
#33638=CARTESIAN_POINT('Ctrl Pts',(4.64357117219061,-4.87429020528853,-2.74406985814738));
#33639=CARTESIAN_POINT('Ctrl Pts',(4.54835473372593,-4.93715636740275,-2.71036603240556));
#33640=CARTESIAN_POINT('Ctrl Pts',(4.5007231232952,-4.96858340495548,-2.69354305704402));
#33641=CARTESIAN_POINT('Ctrl Pts',(4.45307482442137,-5.,-2.67675134594781));
#33642=CARTESIAN_POINT('',(4.45307482442096,-4.81813466520527,-2.99175134594813));
#33643=CARTESIAN_POINT('Origin',(4.45307482442111,-0.181865334794209,5.66850269189656));
#33644=CARTESIAN_POINT('',(4.45307482442111,-0.181865334794209,5.66850269189656));
#33645=CARTESIAN_POINT('',(4.45307482442096,-0.181865334794732,5.66850269189626));
#33646=CARTESIAN_POINT('Ctrl Pts',(4.45307482442111,-0.181865334794216,
5.66850269189656));
#33647=CARTESIAN_POINT('Ctrl Pts',(4.50072369958569,-0.151614623021643,
5.64969075051405));
#33648=CARTESIAN_POINT('Ctrl Pts',(4.54835588590163,-0.121331613566889,
5.63088539794693));
#33649=CARTESIAN_POINT('Ctrl Pts',(4.64357232351274,-0.0607101616775566,
5.59329361772537));
#33650=CARTESIAN_POINT('Ctrl Pts',(4.69115813327592,-0.0303707474635743,
5.57450657478233));
#33651=CARTESIAN_POINT('Ctrl Pts',(4.73872559218025,-2.12704816375314E-15,
5.5557267768221));
#33652=CARTESIAN_POINT('Origin',(4.73872559218025,-4.81140052521338,2.77786338841105));
#33653=CARTESIAN_POINT('',(4.45307482442111,-5.,2.67675134594873));
#33654=CARTESIAN_POINT('Ctrl Pts',(4.45307482442111,-5.,2.67675134594873));
#33655=CARTESIAN_POINT('Ctrl Pts',(4.50072369957508,-4.96858302498895,2.69354326013135));
#33656=CARTESIAN_POINT('Ctrl Pts',(4.54835588589647,-4.93715560720775,2.71036643934055));
#33657=CARTESIAN_POINT('Ctrl Pts',(4.64357232351721,-4.87428944461137,2.74407026658364));
#33658=CARTESIAN_POINT('Ctrl Pts',(4.6911581332779,-4.84284968105536,2.76095144855649));
#33659=CARTESIAN_POINT('Ctrl Pts',(4.73872559218025,-4.81140052521337,2.77786338841105));
#33660=CARTESIAN_POINT('',(4.45307482442096,-4.81813466520527,2.99175134594813));
#33661=CARTESIAN_POINT('Ctrl Pts',(4.73872559218025,-4.81140052521338,2.77786338841104));
#33662=CARTESIAN_POINT('Ctrl Pts',(4.69115755784599,-4.81247894663861,2.81355555799439));
#33663=CARTESIAN_POINT('Ctrl Pts',(4.64357117219958,-4.81357930955884,2.84922421411712));
#33664=CARTESIAN_POINT('Ctrl Pts',(4.54835473372284,-4.8158240213191,2.92051982042641));
#33665=CARTESIAN_POINT('Ctrl Pts',(4.50072312328868,-4.81696841606522,2.95614792099609));
#33666=CARTESIAN_POINT('Ctrl Pts',(4.45307482442137,-4.81813466520499,2.99175134594829));
#33667=CARTESIAN_POINT('',(4.45307482442096,-5.,2.67675134594813));
#33668=CARTESIAN_POINT('Ctrl Pts',(4.44772342888108,-4.83460764645848,2.98224066578723));
#33669=CARTESIAN_POINT('Ctrl Pts',(4.69727026033307,-4.0685083832918,3.42454828160249));
#33670=CARTESIAN_POINT('Ctrl Pts',(4.96928012765321,-2.57903063991063,4.28449865769556));
#33671=CARTESIAN_POINT('Ctrl Pts',(4.78045253748373,-1.18685803776377,5.08826988430348));
#33672=CARTESIAN_POINT('Ctrl Pts',(4.44772342888108,-0.165392353541525,
5.67801337205715));
#33673=CARTESIAN_POINT('Ctrl Pts',(4.5447241499808,-4.82687193937678,2.91411490666184));
#33674=CARTESIAN_POINT('Ctrl Pts',(4.7983881862218,-4.05643946930472,3.36029185661963));
#33675=CARTESIAN_POINT('Ctrl Pts',(5.07815075443907,-2.55113692610128,4.23205467728278));
#33676=CARTESIAN_POINT('Ctrl Pts',(4.8829428649688,-1.13908398007107,5.04508368564026));
#33677=CARTESIAN_POINT('Ctrl Pts',(4.5447241499808,-0.110261569027683,5.63725117364547));
#33678=CARTESIAN_POINT('Ctrl Pts',(4.64172487108053,-4.81913623229508,2.84598914753644));
#33679=CARTESIAN_POINT('Ctrl Pts',(4.89950611211053,-4.04437055531763,3.29603543163677));
#33680=CARTESIAN_POINT('Ctrl Pts',(5.18702138122492,-2.52324321229192,4.17961069686999));
#33681=CARTESIAN_POINT('Ctrl Pts',(4.98543319245386,-1.09130992237837,5.00189748697704));
#33682=CARTESIAN_POINT('Ctrl Pts',(4.64172487108053,-0.0551307845138405,
5.59648897523378));
#33683=CARTESIAN_POINT('Ctrl Pts',(4.73872559218025,-4.81140052521338,2.77786338841104));
#33684=CARTESIAN_POINT('Ctrl Pts',(5.00062403799926,-4.03230164133055,3.2317790066539));
#33685=CARTESIAN_POINT('Ctrl Pts',(5.29589200801077,-2.49534949848256,4.12716671645721));
#33686=CARTESIAN_POINT('Ctrl Pts',(5.08792351993893,-1.04353586468567,4.95871128831382));
#33687=CARTESIAN_POINT('Ctrl Pts',(4.73872559218025,1.94289029309402E-15,
5.5557267768221));
#33688=CARTESIAN_POINT('Ctrl Pts',(4.45307670887187,-0.181867076559572,
5.66850168628786));
#33689=CARTESIAN_POINT('Ctrl Pts',(4.78160975160098,-1.1954229142106,5.08332495058132));
#33690=CARTESIAN_POINT('Ctrl Pts',(4.96786706546316,-2.57932900588259,4.28432639602133));
#33691=CARTESIAN_POINT('Ctrl Pts',(4.69893917059593,-4.05934677490055,3.42983773867339));
#33692=CARTESIAN_POINT('Ctrl Pts',(4.45307570990783,-4.81813302518876,2.9917522928121));
#33693=CARTESIAN_POINT('Origin',(0.,-4.90906733260264,2.83425134594813));
#33694=CARTESIAN_POINT('',(0.528943702130891,-4.81813466520527,2.99175134594813));
#33695=CARTESIAN_POINT('',(0.528943702130891,-5.,2.67675134594813));
#33696=CARTESIAN_POINT('Ctrl Pts',(0.528943702130891,-4.81813466520527,
2.99175134594813));
#33697=CARTESIAN_POINT('Ctrl Pts',(0.525532604501329,-4.90906733260263,
2.83425134594813));
#33698=CARTESIAN_POINT('Ctrl Pts',(0.528943702130891,-5.,2.67675134594813));
#33699=CARTESIAN_POINT('',(0.,-5.,2.67675134594813));
#33700=CARTESIAN_POINT('',(0.,-4.81813466520527,2.99175134594813));
#33701=CARTESIAN_POINT('Ctrl Pts',(4.44772342888108,-5.,-2.69577270626992));
#33702=CARTESIAN_POINT('Ctrl Pts',(4.78045253748373,-5.,-1.51628573076256));
#33703=CARTESIAN_POINT('Ctrl Pts',(4.96948022596782,-5.,0.0912172907134438));
#33704=CARTESIAN_POINT('Ctrl Pts',(4.69727026033307,-5.,1.8111574746394));
#33705=CARTESIAN_POINT('Ctrl Pts',(4.44772342888108,-5.,2.69577270626992));
#33706=CARTESIAN_POINT('Ctrl Pts',(4.5447241499808,-4.93713350840446,-2.72313626698363));
#33707=CARTESIAN_POINT('Ctrl Pts',(4.8829428649688,-4.93871262601842,-1.53606617903469));
#33708=CARTESIAN_POINT('Ctrl Pts',(5.07834742005573,-4.94063410426251,0.0932810725788998));
#33709=CARTESIAN_POINT('Ctrl Pts',(4.7983881862218,-4.93831784661493,1.83283370102193));
#33710=CARTESIAN_POINT('Ctrl Pts',(4.5447241499808,-4.93713350840446,2.72313626698363));
#33711=CARTESIAN_POINT('Ctrl Pts',(4.64172487108053,-4.87426701680892,-2.75049982769734));
#33712=CARTESIAN_POINT('Ctrl Pts',(4.98543319245387,-4.87742525203684,-1.55584662730683));
#33713=CARTESIAN_POINT('Ctrl Pts',(5.18721461414363,-4.88126820852503,0.0953448544443579));
#33714=CARTESIAN_POINT('Ctrl Pts',(4.89950611211053,-4.87663569322986,1.85450992740445));
#33715=CARTESIAN_POINT('Ctrl Pts',(4.64172487108053,-4.87426701680892,2.75049982769734));
#33716=CARTESIAN_POINT('Ctrl Pts',(4.73872559218025,-4.81140052521337,-2.77786338841105));
#33717=CARTESIAN_POINT('Ctrl Pts',(5.08792351993893,-4.81613787805526,-1.57562707557896));
#33718=CARTESIAN_POINT('Ctrl Pts',(5.29608180823153,-4.82190231278754,0.0974086363098129));
#33719=CARTESIAN_POINT('Ctrl Pts',(5.00062403799926,-4.81495353984479,1.87618615378698));
#33720=CARTESIAN_POINT('Ctrl Pts',(4.73872559218025,-4.81140052521337,2.77786338841105));
#33721=CARTESIAN_POINT('Ctrl Pts',(4.45307572309967,-5.,2.67674944962107));
#33722=CARTESIAN_POINT('Ctrl Pts',(4.6989403977156,-5.,1.80057831867945));
#33723=CARTESIAN_POINT('Ctrl Pts',(4.96806593665806,-5.,0.091562055880635));
#33724=CARTESIAN_POINT('Ctrl Pts',(4.78161097872072,-5.,-1.50639610513643));
#33725=CARTESIAN_POINT('Ctrl Pts',(4.45307671877196,-5.,-2.67674933668171));
#33726=CARTESIAN_POINT('Origin',(0.,-1.56125112837913E-16,5.66850269189626));
#33727=CARTESIAN_POINT('',(0.528943702130891,0.181865334794732,5.66850269189626));
#33728=CARTESIAN_POINT('',(0.528943702130891,-0.181865334794732,5.66850269189626));
#33729=CARTESIAN_POINT('Ctrl Pts',(0.528943702130891,0.181865334794732,
5.66850269189626));
#33730=CARTESIAN_POINT('Ctrl Pts',(0.525532604501329,-1.14491749414469E-15,
5.66850269189626));
#33731=CARTESIAN_POINT('Ctrl Pts',(0.528943702130891,-0.181865334794732,
5.66850269189626));
#33732=CARTESIAN_POINT('',(0.,-0.181865334794732,5.66850269189626));
#33733=CARTESIAN_POINT('',(0.,0.181865334794732,5.66850269189626));
#33734=CARTESIAN_POINT('Origin',(0.,-4.90906733260263,-2.83425134594813));
#33735=CARTESIAN_POINT('',(0.52894370213089,-5.,-2.67675134594813));
#33736=CARTESIAN_POINT('',(0.528943702130891,-4.81813466520527,-2.99175134594813));
#33737=CARTESIAN_POINT('Ctrl Pts',(0.52894370213089,-5.,-2.67675134594813));
#33738=CARTESIAN_POINT('Ctrl Pts',(0.525532604501329,-4.90906733260263,
-2.83425134594813));
#33739=CARTESIAN_POINT('Ctrl Pts',(0.528943702130891,-4.81813466520527,
-2.99175134594813));
#33740=CARTESIAN_POINT('',(0.,-4.81813466520527,-2.99175134594813));
#33741=CARTESIAN_POINT('',(0.,-5.,-2.67675134594813));
#33742=CARTESIAN_POINT('Ctrl Pts',(4.44772342888108,-0.165392353541525,
-5.67801337205715));
#33743=CARTESIAN_POINT('Ctrl Pts',(4.69727026033307,-0.931491616708205,
-5.2357057562419));
#33744=CARTESIAN_POINT('Ctrl Pts',(4.96928012765321,-2.42096936008937,-4.37575538014882));
#33745=CARTESIAN_POINT('Ctrl Pts',(4.78045253748373,-3.81314196223624,-3.57198415354091));
#33746=CARTESIAN_POINT('Ctrl Pts',(4.44772342888108,-4.83460764645847,-2.98224066578724));
#33747=CARTESIAN_POINT('Ctrl Pts',(4.5447241499808,-0.110261569027682,-5.63725117364547));
#33748=CARTESIAN_POINT('Ctrl Pts',(4.7983881862218,-0.881878377310218,-5.19312555764156));
#33749=CARTESIAN_POINT('Ctrl Pts',(5.07815075443906,-2.389498397681,-4.32537672517764));
#33750=CARTESIAN_POINT('Ctrl Pts',(4.8829428649688,-3.79962864594736,-3.50901750660556));
#33751=CARTESIAN_POINT('Ctrl Pts',(4.5447241499808,-4.82687193937677,-2.91411490666184));
#33752=CARTESIAN_POINT('Ctrl Pts',(4.64172487108053,-0.0551307845138397,
-5.59648897523378));
#33753=CARTESIAN_POINT('Ctrl Pts',(4.89950611211053,-0.832265137912234,
-5.15054535904123));
#33754=CARTESIAN_POINT('Ctrl Pts',(5.18702138122492,-2.35802743527264,-4.27499807020645));
#33755=CARTESIAN_POINT('Ctrl Pts',(4.98543319245386,-3.78611532965848,-3.44605085967021));
#33756=CARTESIAN_POINT('Ctrl Pts',(4.64172487108053,-4.81913623229507,-2.84598914753644));
#33757=CARTESIAN_POINT('Ctrl Pts',(4.73872559218025,2.80742846517038E-15,
-5.5557267768221));
#33758=CARTESIAN_POINT('Ctrl Pts',(5.00062403799926,-0.782651898514247,
-5.10796516044089));
#33759=CARTESIAN_POINT('Ctrl Pts',(5.29589200801077,-2.32655647286427,-4.22461941523526));
#33760=CARTESIAN_POINT('Ctrl Pts',(5.08792351993893,-3.7726020133696,-3.38308421273486));
#33761=CARTESIAN_POINT('Ctrl Pts',(4.73872559218025,-4.81140052521337,-2.77786338841105));
#33762=CARTESIAN_POINT('Ctrl Pts',(4.45307670887188,-4.81813292344042,-2.99175235155653));
#33763=CARTESIAN_POINT('Ctrl Pts',(4.78160975160098,-3.8045770857894,-3.57692908726306));
#33764=CARTESIAN_POINT('Ctrl Pts',(4.96786706546316,-2.42067099411741,-4.37592764182305));
#33765=CARTESIAN_POINT('Ctrl Pts',(4.69893917059593,-0.940653225099448,
-5.230416299171));
#33766=CARTESIAN_POINT('Ctrl Pts',(4.45307570990783,-0.181866974811239,
-5.66850174503229));
#33767=CARTESIAN_POINT('Origin',(0.,4.90906733260264,2.83425134594813));
#33768=CARTESIAN_POINT('',(0.528943702130891,5.,2.67675134594813));
#33769=CARTESIAN_POINT('',(0.528943702130891,4.81813466520527,2.99175134594813));
#33770=CARTESIAN_POINT('Ctrl Pts',(0.528943702130891,5.,2.67675134594813));
#33771=CARTESIAN_POINT('Ctrl Pts',(0.525532604501329,4.90906733260263,2.83425134594813));
#33772=CARTESIAN_POINT('Ctrl Pts',(0.528943702130891,4.81813466520527,2.99175134594813));
#33773=CARTESIAN_POINT('',(0.,4.81813466520527,2.99175134594813));
#33774=CARTESIAN_POINT('',(0.,5.,2.67675134594813));
#33775=CARTESIAN_POINT('Origin',(0.,-1.37043154602168E-15,-5.66850269189626));
#33776=CARTESIAN_POINT('',(0.528943702130891,-0.181865334794732,-5.66850269189626));
#33777=CARTESIAN_POINT('',(0.528943702130891,0.181865334794731,-5.66850269189626));
#33778=CARTESIAN_POINT('Ctrl Pts',(0.528943702130891,-0.181865334794732,
-5.66850269189626));
#33779=CARTESIAN_POINT('Ctrl Pts',(0.525532604501329,3.46944695195361E-17,
-5.66850269189626));
#33780=CARTESIAN_POINT('Ctrl Pts',(0.528943702130891,0.181865334794731,
-5.66850269189626));
#33781=CARTESIAN_POINT('',(0.,0.18186533479473,-5.66850269189626));
#33782=CARTESIAN_POINT('',(0.,-0.181865334794733,-5.66850269189626));
#33783=CARTESIAN_POINT('Origin',(0.,4.90906733260263,-2.83425134594813));
#33784=CARTESIAN_POINT('',(0.528943702130891,4.81813466520527,-2.99175134594813));
#33785=CARTESIAN_POINT('',(0.52894370213089,5.,-2.67675134594813));
#33786=CARTESIAN_POINT('Ctrl Pts',(0.528943702130891,4.81813466520527,-2.99175134594813));
#33787=CARTESIAN_POINT('Ctrl Pts',(0.525532604501329,4.90906733260263,-2.83425134594813));
#33788=CARTESIAN_POINT('Ctrl Pts',(0.52894370213089,5.,-2.67675134594813));
#33789=CARTESIAN_POINT('',(0.,5.,-2.67675134594813));
#33790=CARTESIAN_POINT('',(0.,4.81813466520527,-2.99175134594813));
#33791=CARTESIAN_POINT('Origin',(0.,5.,2.88675134594813));
#33792=CARTESIAN_POINT('Ctrl Pts',(0.528943702130891,4.81813466520527,2.99175134594813));
#33793=CARTESIAN_POINT('Ctrl Pts',(-0.209998305499054,2.5,4.33012701892219));
#33794=CARTESIAN_POINT('Ctrl Pts',(0.528943702130891,0.181865334794731,
5.66850269189626));
#33795=CARTESIAN_POINT('Origin',(0.,5.,-2.88675134594813));
#33796=CARTESIAN_POINT('Ctrl Pts',(0.52894370213089,5.,-2.67675134594813));
#33797=CARTESIAN_POINT('Ctrl Pts',(-0.209998305499052,5.,-5.55111512312578E-16));
#33798=CARTESIAN_POINT('Ctrl Pts',(0.528943702130891,5.,2.67675134594813));
#33799=CARTESIAN_POINT('Origin',(0.,-1.06057523872491E-15,-5.77350269189626));
#33800=CARTESIAN_POINT('Ctrl Pts',(0.528943702130891,0.181865334794731,
-5.66850269189626));
#33801=CARTESIAN_POINT('Ctrl Pts',(-0.209998305499051,2.5,-4.33012701892219));
#33802=CARTESIAN_POINT('Ctrl Pts',(0.528943702130891,4.81813466520527,-2.99175134594813));
#33803=CARTESIAN_POINT('Origin',(0.377062317719749,0.,0.));
#33804=CARTESIAN_POINT('',(0.136226494320606,-5.,-3.68823841089113E-16));
#33805=CARTESIAN_POINT('',(0.377062317719749,-5.41175134594813,-6.62748396359676E-16));
#33806=CARTESIAN_POINT('Ctrl Pts',(0.528943702130891,-5.,2.67675134594813));
#33807=CARTESIAN_POINT('Ctrl Pts',(0.136226494320606,-5.,1.25416837769224));
#33808=CARTESIAN_POINT('Ctrl Pts',(0.136226494320606,-5.,-1.25324282604549E-16));
#33809=CARTESIAN_POINT('Ctrl Pts',(0.528943702130891,-0.181865334794732,
5.66850269189626));
#33810=CARTESIAN_POINT('Ctrl Pts',(-0.209998305499052,-2.5,4.33012701892219));
#33811=CARTESIAN_POINT('Ctrl Pts',(0.528943702130891,-4.81813466520527,
2.99175134594813));
#33812=CARTESIAN_POINT('Ctrl Pts',(0.528943702130891,-4.81813466520527,
-2.99175134594813));
#33813=CARTESIAN_POINT('Ctrl Pts',(-0.209998305499052,-2.5,-4.33012701892219));
#33814=CARTESIAN_POINT('Ctrl Pts',(0.528943702130891,-0.181865334794732,
-5.66850269189626));
#33815=CARTESIAN_POINT('Ctrl Pts',(0.136226494320606,-5.,-1.25324282604549E-16));
#33816=CARTESIAN_POINT('Ctrl Pts',(0.136226494320606,-5.,-1.25416837769224));
#33817=CARTESIAN_POINT('Ctrl Pts',(0.52894370213089,-5.,-2.67675134594813));
#33818=CARTESIAN_POINT('Origin',(0.,-5.,-2.88675134594813));
#33819=CARTESIAN_POINT('Origin',(0.,-5.,2.88675134594813));
#33820=CARTESIAN_POINT('Origin',(0.,3.53525079574969E-16,5.77350269189626));
#38509=UNCERTAINTY_MEASURE_WITH_UNIT(LENGTH_MEASURE(0.01),#38529,
'DISTANCE_ACCURACY_VALUE',
'Maximum model space distance between geometric entities at asserted c
onnectivities');
#38514=UNCERTAINTY_MEASURE_WITH_UNIT(LENGTH_MEASURE(0.01),#38529,
'DISTANCE_ACCURACY_VALUE',
'Maximum model space distance between geometric entities at asserted c
onnectivities');
#38523=(
GEOMETRIC_REPRESENTATION_CONTEXT(3)
GLOBAL_UNCERTAINTY_ASSIGNED_CONTEXT((#38509))
GLOBAL_UNIT_ASSIGNED_CONTEXT((#38529,#38531,#38532))
REPRESENTATION_CONTEXT('','3D')
);
#38528=(
GEOMETRIC_REPRESENTATION_CONTEXT(3)
GLOBAL_UNCERTAINTY_ASSIGNED_CONTEXT((#38514))
GLOBAL_UNIT_ASSIGNED_CONTEXT((#38529,#38531,#38532))
REPRESENTATION_CONTEXT('','3D')
);
#38529=(
LENGTH_UNIT()
NAMED_UNIT(*)
SI_UNIT(.MILLI.,.METRE.)
);
#38531=(
NAMED_UNIT(*)
PLANE_ANGLE_UNIT()
SI_UNIT($,.RADIAN.)
);
#38532=(
NAMED_UNIT(*)
SI_UNIT($,.STERADIAN.)
SOLID_ANGLE_UNIT()
);
#38541=SHAPE_DEFINITION_REPRESENTATION(#38554,#38583);
#38554=PRODUCT_DEFINITION_SHAPE('',$,#38597);
#38583=SHAPE_REPRESENTATION('',(#18722),#38523);
#38588=PRODUCT_DEFINITION_CONTEXT('part definition',#38629,'design');
#38597=PRODUCT_DEFINITION('2026-10-20-13-39-09-546',
'08_ISO_4032_Nut_M6',#38610,#38588);
#38610=PRODUCT_DEFINITION_FORMATION('',$,#38639);
#38629=APPLICATION_CONTEXT(
'Core Data for Automotive Mechanical Design Process');
#38630=PRODUCT_CONTEXT('part definition',#38629,'mechanical');
#38639=PRODUCT('2026-10-20-13-39-09-546','08_ISO_4032_Nut_M6',$,(#38630));
#38707=COLOUR_RGB('Black',0.12,0.14,0.17);
#38708=FILL_AREA_STYLE_COLOUR('',#38707);
#38709=FILL_AREA_STYLE('',(#38708));
#38710=SURFACE_STYLE_FILL_AREA(#38709);
#38711=SURFACE_SIDE_STYLE('',(#38710));
#38712=SURFACE_STYLE_USAGE(.BOTH.,#38711);
#38713=PRESENTATION_STYLE_ASSIGNMENT((#38712));
ENDSEC;
END-ISO-10303-21;
